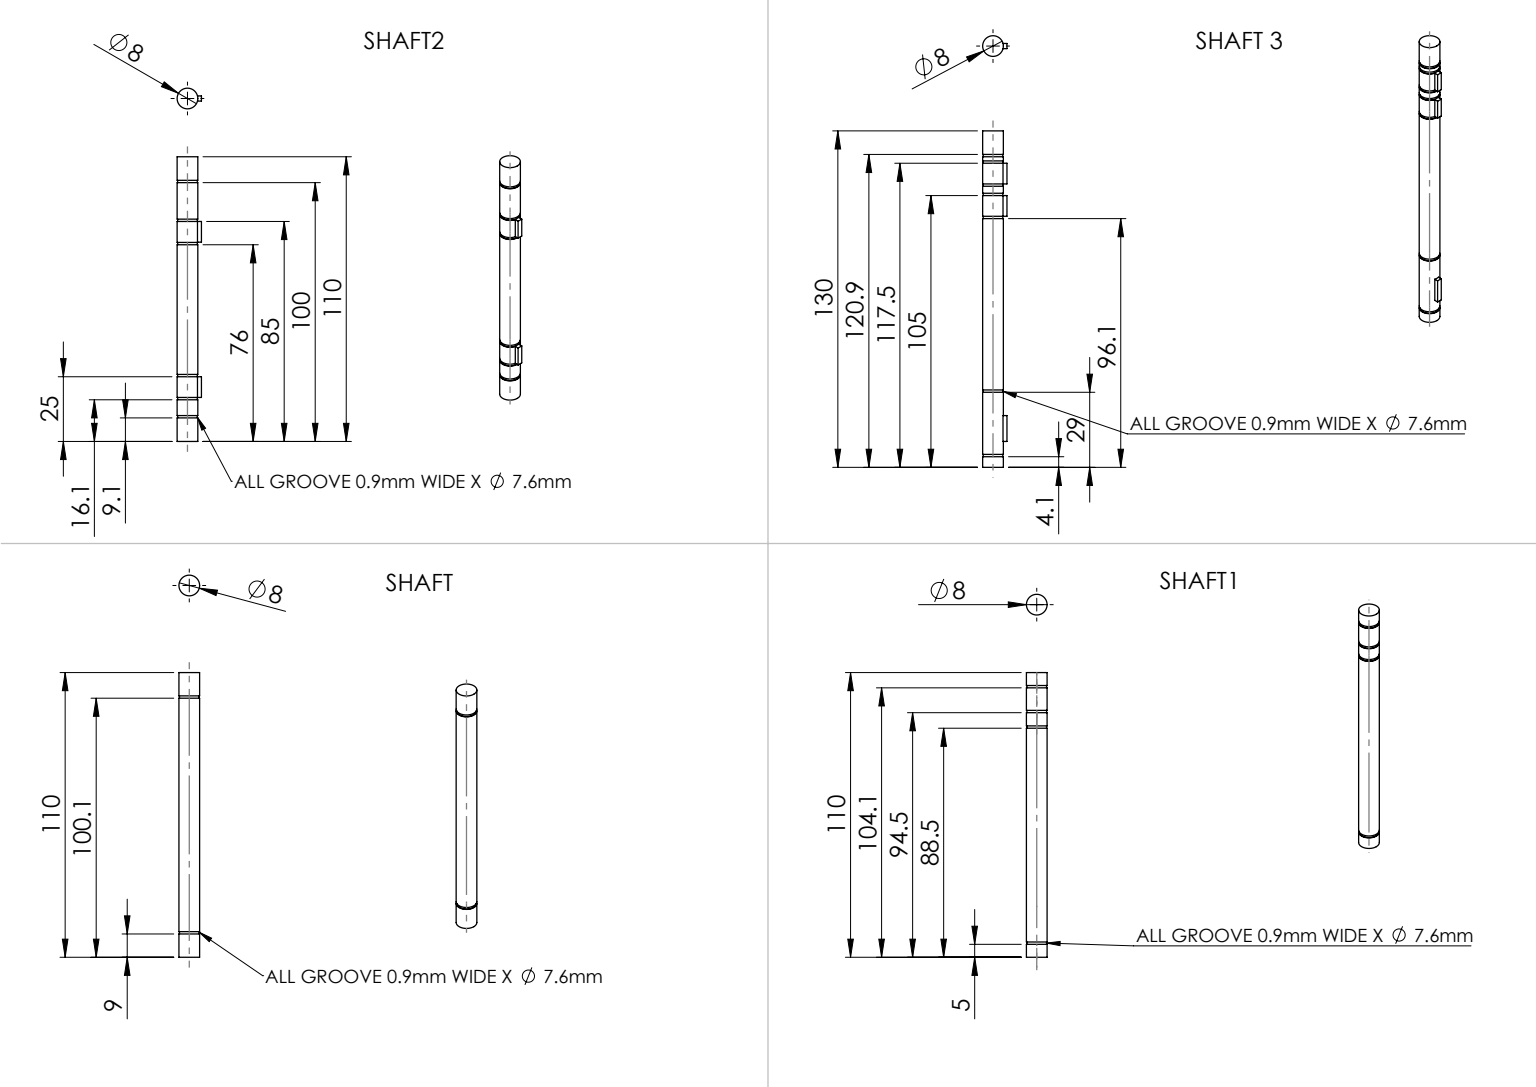
ISO-10303-21;
HEADER;
FILE_DESCRIPTION (('STEP AP214'),
    '1' );
FILE_NAME ('shaft2.step',
    '2026-09-28T15:49:00',
    ( '' ),
    ( '' ),
    'SwSTEP 2.0',
    'SolidWorks 2026',
    '' );
FILE_SCHEMA (( 'AUTOMOTIVE_DESIGN' ));
ENDSEC;

DATA;
#32=ORIENTED_EDGE ( 'NONE', *, *, #23830, .T. ) ;
#40=FACE_OUTER_BOUND ( 'NONE', #7039, .T. ) ;
#47=DIRECTION ( 'NONE',  ( 0.000000000000000000, 0.000000000000000000, -1.000000000000000000 ) ) ;
#82=CARTESIAN_POINT ( 'NONE',  ( -3.799999999999999822, 4.382607293638566128E-16, -21.89999999999999858 ) ) ;
#98=( GEOMETRIC_REPRESENTATION_CONTEXT ( 3 ) GLOBAL_UNCERTAINTY_ASSIGNED_CONTEXT ( ( #24807 ) ) GLOBAL_UNIT_ASSIGNED_CONTEXT ( ( #15841, #16194, #16020 ) ) REPRESENTATION_CONTEXT ( 'NONE', 'WORKASPACE' ) );
#117=DIRECTION ( 'NONE',  ( -1.000000000000000000, 0.000000000000000000, 0.000000000000000000 ) ) ;
#178=CIRCLE ( 'NONE', #22577, 4.000000000000000000 ) ;
#185=VERTEX_POINT ( 'NONE', #4789 ) ;
#210=CARTESIAN_POINT ( 'NONE',  ( 5.400000000000015454, -1.000000000000002220, -22.00000000000000000 ) ) ;
#255=CARTESIAN_POINT ( 'NONE',  ( 0.000000000000000000, -2.710505431213761085E-17, -45.89999999999999858 ) ) ;
#260=ORIENTED_EDGE ( 'NONE', *, *, #3308, .F. ) ;
#266=ORIENTED_EDGE ( 'NONE', *, *, #9713, .F. ) ;
#278=VECTOR ( 'NONE', #10313, 1000.000000000000000 ) ;
#308=ORIENTED_EDGE ( 'NONE', *, *, #26431, .T. ) ;
#342=VERTEX_POINT ( 'NONE', #32678 ) ;
#351=DIRECTION ( 'NONE',  ( -1.000000000000000000, 0.000000000000000000, 0.000000000000000000 ) ) ;
#427=DIRECTION ( 'NONE',  ( 0.000000000000000000, 0.000000000000000000, -1.000000000000000000 ) ) ;
#440=VERTEX_POINT ( 'NONE', #35039 ) ;
#452=ORIENTED_EDGE ( 'NONE', *, *, #14571, .F. ) ;
#462=CARTESIAN_POINT ( 'NONE',  ( 0.000000000000000000, -2.710505431213761085E-17, -21.89999999999999858 ) ) ;
#493=DIRECTION ( 'NONE',  ( 1.000000000000000000, 0.000000000000000000, 0.000000000000000000 ) ) ;
#496=EDGE_CURVE ( 'NONE', #185, #4943, #8530, .T. ) ;
#500=ORIENTED_EDGE ( 'NONE', *, *, #33503, .T. ) ;
#516=FACE_BOUND ( 'NONE', #19608, .T. ) ;
#542=VERTEX_POINT ( 'NONE', #3500 ) ;
#583=DIRECTION ( 'NONE',  ( -1.000000000000000000, 0.000000000000000000, 0.000000000000000000 ) ) ;
#606=CARTESIAN_POINT ( 'NONE',  ( 6.071532165918824830E-15, 1.000000000000000000, 38.00000000000000000 ) ) ;
#619=EDGE_LOOP ( 'NONE', ( #5194, #17904, #27219, #22825 ) ) ;
#628=EDGE_CURVE ( 'NONE', #13726, #1603, #27780, .T. ) ;
#657=EDGE_CURVE ( 'NONE', #5410, #7912, #11948, .T. ) ;
#751=VERTEX_POINT ( 'NONE', #15513 ) ;
#763=DIRECTION ( 'NONE',  ( -0.000000000000000000, 0.000000000000000000, -1.000000000000000000 ) ) ;
#798=DIRECTION ( 'NONE',  ( -1.000000000000000000, 0.000000000000000000, 0.000000000000000000 ) ) ;
#813=PRESENTATION_STYLE_ASSIGNMENT (( #32934 ) ) ;
#825=ORIENTED_EDGE ( 'NONE', *, *, #30231, .F. ) ;
#844=PLANE ( 'NONE',  #8243 ) ;
#853=DIRECTION ( 'NONE',  ( -0.000000000000000000, 0.000000000000000000, -1.000000000000000000 ) ) ;
#880=VECTOR ( 'NONE', #6059, 1000.000000000000000 ) ;
#908=VERTEX_POINT ( 'NONE', #15691 ) ;
#960=LINE ( 'NONE', #1142, #3147 ) ;
#991=CARTESIAN_POINT ( 'NONE',  ( 0.000000000000000000, -2.710505431213761085E-17, 55.00000000000000000 ) ) ;
#1001=VECTOR ( 'NONE', #23243, 1000.000000000000000 ) ;
#1044=ORIENTED_EDGE ( 'NONE', *, *, #17234, .T. ) ;
#1056=CARTESIAN_POINT ( 'NONE',  ( -4.000000000000000000, -2.710505431213761085E-17, -20.99999999999999645 ) ) ;
#1068=ORIENTED_EDGE ( 'NONE', *, *, #2171, .T. ) ;
#1072=ORIENTED_EDGE ( 'NONE', *, *, #10606, .F. ) ;
#1142=CARTESIAN_POINT ( 'NONE',  ( 5.400000000000015454, -1.000000000000002220, 38.00000000000000000 ) ) ;
#1161=ORIENTED_EDGE ( 'NONE', *, *, #13775, .T. ) ;
#1195=ORIENTED_EDGE ( 'NONE', *, *, #24033, .T. ) ;
#1209=DIRECTION ( 'NONE',  ( -1.000000000000000000, 0.000000000000000000, 0.000000000000000000 ) ) ;
#1266=EDGE_LOOP ( 'NONE', ( #9909, #9614 ) ) ;
#1268=CARTESIAN_POINT ( 'NONE',  ( 5.400000000000015454, -1.000000000000002220, 38.00000000000000000 ) ) ;
#1317=VERTEX_POINT ( 'NONE', #31534 ) ;
#1353=UNCERTAINTY_MEASURE_WITH_UNIT (LENGTH_MEASURE( 1.000000000000000082E-05 ), #3538, 'distance_accuracy_value', 'NONE');
#1355=EDGE_LOOP ( 'NONE', ( #23025, #6634 ) ) ;
#1381=ORIENTED_EDGE ( 'NONE', *, *, #35324, .T. ) ;
#1383=CARTESIAN_POINT ( 'NONE',  ( -4.000000000000000000, -2.710505431213761085E-17, -30.00000000000000711 ) ) ;
#1402=DIRECTION ( 'NONE',  ( 0.000000000000000000, 0.000000000000000000, -1.000000000000000000 ) ) ;
#1407=CARTESIAN_POINT ( 'NONE',  ( 0.000000000000000000, -2.710505431213761085E-17, -45.00000000000000000 ) ) ;
#1426=CIRCLE ( 'NONE', #24430, 4.000000000000000000 ) ;
#1443=LINE ( 'NONE', #17456, #9565 ) ;
#1459=AXIS2_PLACEMENT_3D ( 'NONE', #33980, #25881, #34827 ) ;
#1469=ORIENTED_EDGE ( 'NONE', *, *, #628, .F. ) ;
#1480=DIRECTION ( 'NONE',  ( 0.000000000000000000, 0.000000000000000000, -1.000000000000000000 ) ) ;
#1503=FACE_OUTER_BOUND ( 'NONE', #12935, .T. ) ;
#1586=ADVANCED_FACE ( 'NONE', ( #16721, #16553 ), #14543, .T. ) ;
#1589=VECTOR ( 'NONE', #10467, 1000.000000000000000 ) ;
#1590=DIRECTION ( 'NONE',  ( 0.000000000000000000, 0.000000000000000000, 1.000000000000000000 ) ) ;
#1592=LINE ( 'NONE', #20641, #29686 ) ;
#1603=VERTEX_POINT ( 'NONE', #14378 ) ;
#1615=CARTESIAN_POINT ( 'NONE',  ( 0.000000000000000000, -2.710505431213761085E-17, 45.00000000000000000 ) ) ;
#1632=FACE_OUTER_BOUND ( 'NONE', #3397, .T. ) ;
#1636=DIRECTION ( 'NONE',  ( 0.000000000000000000, 0.000000000000000000, -1.000000000000000000 ) ) ;
#1656=VERTEX_POINT ( 'NONE', #24846 ) ;
#1666=AXIS2_PLACEMENT_3D ( 'NONE', #8199, #16112, #18830 ) ;
#1816=CARTESIAN_POINT ( 'NONE',  ( 0.000000000000000000, -2.710505431213761085E-17, 38.90000000000000568 ) ) ;
#1886=AXIS2_PLACEMENT_3D ( 'NONE', #15897, #7452, #7275 ) ;
#1914=DIRECTION ( 'NONE',  ( -0.000000000000000000, 0.000000000000000000, -1.000000000000000000 ) ) ;
#1927=ORIENTED_EDGE ( 'NONE', *, *, #25819, .F. ) ;
#1951=ADVANCED_FACE ( 'NONE', ( #32372, #32541 ), #35096, .F. ) ;
#1972=ORIENTED_EDGE ( 'NONE', *, *, #26406, .F. ) ;
#2019=( NAMED_UNIT ( * ) PLANE_ANGLE_UNIT ( ) SI_UNIT ( $, .RADIAN. ) );
#2103=DIRECTION ( 'NONE',  ( 1.000000000000000000, 0.000000000000000000, 0.000000000000000000 ) ) ;
#2109=DIRECTION ( 'NONE',  ( 1.000000000000000000, 0.000000000000000000, 0.000000000000000000 ) ) ;
#2124=VECTOR ( 'NONE', #11080, 1000.000000000000000 ) ;
#2160=ORIENTED_EDGE ( 'NONE', *, *, #21209, .T. ) ;
#2171=EDGE_CURVE ( 'NONE', #13101, #10171, #22102, .T. ) ;
#2187=CARTESIAN_POINT ( 'NONE',  ( -3.799999999999999822, 4.382607293638566128E-16, 38.00000000000000711 ) ) ;
#2192=DIRECTION ( 'NONE',  ( -1.000000000000000000, 1.110223024625156540E-16, 0.000000000000000000 ) ) ;
#2240=LINE ( 'NONE', #24180, #6682 ) ;
#2272=ORIENTED_EDGE ( 'NONE', *, *, #11488, .F. ) ;
#2281=CARTESIAN_POINT ( 'NONE',  ( 0.000000000000000000, -2.710505431213761085E-17, 45.89999999999999858 ) ) ;
#2288=VERTEX_POINT ( 'NONE', #17558 ) ;
#2313=DIRECTION ( 'NONE',  ( 1.000000000000000000, -1.110223024625156540E-16, 0.000000000000000000 ) ) ;
#2325=CARTESIAN_POINT ( 'NONE',  ( 3.872983346207429900, -1.000000000000003553, -30.00000000000000711 ) ) ;
#2330=VERTEX_POINT ( 'NONE', #28745 ) ;
#2342=EDGE_LOOP ( 'NONE', ( #31787, #21630, #16161, #3142, #11858 ) ) ;
#2389=DIRECTION ( 'NONE',  ( -0.000000000000000000, 0.000000000000000000, -1.000000000000000000 ) ) ;
#2447=EDGE_CURVE ( 'NONE', #26362, #542, #27119, .T. ) ;
#2545=CIRCLE ( 'NONE', #18605, 3.799999999999999822 ) ;
#2556=ORIENTED_EDGE ( 'NONE', *, *, #17988, .F. ) ;
#2559=SHAPE_REPRESENTATION_RELATIONSHIP ( 'NONE' , 'NONE' ,  #5681, #8640 ) ;
#2582=CIRCLE ( 'NONE', #29610, 4.000000000000000000 ) ;
#2638=ORIENTED_EDGE ( 'NONE', *, *, #16294, .T. ) ;
#2640=ORIENTED_EDGE ( 'NONE', *, *, #29026, .T. ) ;
#2644=ORIENTED_EDGE ( 'NONE', *, *, #496, .F. ) ;
#2660=EDGE_CURVE ( 'NONE', #15153, #17557, #13600, .T. ) ;
#2686=CIRCLE ( 'NONE', #22185, 3.799999999999999822 ) ;
#2770=CARTESIAN_POINT ( 'NONE',  ( 0.000000000000000000, -2.710505431213761085E-17, 38.00000000000000711 ) ) ;
#2821=VECTOR ( 'NONE', #6341, 1000.000000000000000 ) ;
#2871=ORIENTED_EDGE ( 'NONE', *, *, #30764, .F. ) ;
#2885=FACE_BOUND ( 'NONE', #33804, .T. ) ;
#2886=DIRECTION ( 'NONE',  ( 0.000000000000000000, 0.000000000000000000, -1.000000000000000000 ) ) ;
#2902=EDGE_LOOP ( 'NONE', ( #9794, #22603, #23283, #8221 ) ) ;
#2907=EDGE_LOOP ( 'NONE', ( #5346, #10050 ) ) ;
#2959=CARTESIAN_POINT ( 'NONE',  ( 3.799999999999999822, 4.382607293638566128E-16, 45.89999999999999858 ) ) ;
#2979=DIRECTION ( 'NONE',  ( 0.000000000000000000, 0.000000000000000000, 1.000000000000000000 ) ) ;
#3015=DIRECTION ( 'NONE',  ( -1.000000000000000000, 1.110223024625156540E-16, 0.000000000000000000 ) ) ;
#3053=ORIENTED_EDGE ( 'NONE', *, *, #8030, .T. ) ;
#3056=DIRECTION ( 'NONE',  ( 0.000000000000000000, 0.000000000000000000, 1.000000000000000000 ) ) ;
#3073=CIRCLE ( 'NONE', #23781, 3.799999999999999822 ) ;
#3142=ORIENTED_EDGE ( 'NONE', *, *, #28661, .T. ) ;
#3147=VECTOR ( 'NONE', #25455, 1000.000000000000000 ) ;
#3151=FACE_OUTER_BOUND ( 'NONE', #30786, .T. ) ;
#3240=ORIENTED_EDGE ( 'NONE', *, *, #31686, .T. ) ;
#3251=ORIENTED_EDGE ( 'NONE', *, *, #9751, .T. ) ;
#3308=EDGE_CURVE ( 'NONE', #13350, #4520, #28897, .T. ) ;
#3310=LINE ( 'NONE', #8861, #35043 ) ;
#3315=CARTESIAN_POINT ( 'NONE',  ( 3.872983346207429900, -1.000000000000003553, 55.00000000000000000 ) ) ;
#3318=CIRCLE ( 'NONE', #23430, 4.000000000000000000 ) ;
#3397=EDGE_LOOP ( 'NONE', ( #19722, #11550, #20094, #1381 ) ) ;
#3437=CARTESIAN_POINT ( 'NONE',  ( 0.000000000000000000, -2.710505431213761085E-17, 55.00000000000000000 ) ) ;
#3452=DIRECTION ( 'NONE',  ( -0.000000000000000000, 0.000000000000000000, -1.000000000000000000 ) ) ;
#3462=VERTEX_POINT ( 'NONE', #30278 ) ;
#3485=ORIENTED_EDGE ( 'NONE', *, *, #23597, .F. ) ;
#3500=CARTESIAN_POINT ( 'NONE',  ( 3.872983346207416133, 1.000000000000001110, -29.99999999999999289 ) ) ;
#3501=ORIENTED_EDGE ( 'NONE', *, *, #30231, .T. ) ;
#3502=CARTESIAN_POINT ( 'NONE',  ( 5.400000000000015454, -1.000000000000002220, 30.00000000000000000 ) ) ;
#3513=EDGE_LOOP ( 'NONE', ( #35507, #10361 ) ) ;
#3529=DIRECTION ( 'NONE',  ( -1.000000000000000000, 0.000000000000000000, 0.000000000000000000 ) ) ;
#3534=DIRECTION ( 'NONE',  ( 0.000000000000000000, 0.000000000000000000, 1.000000000000000000 ) ) ;
#3538=( LENGTH_UNIT ( ) NAMED_UNIT ( * ) SI_UNIT ( .MILLI., .METRE. ) );
#3542=LINE ( 'NONE', #14490, #19352 ) ;
#3566=CARTESIAN_POINT ( 'NONE',  ( 3.799999999999999822, -2.710505431213761085E-17, -30.00000000000000711 ) ) ;
#3582=STYLED_ITEM ( 'NONE', ( #813 ), #22482 ) ;
#3641=DIRECTION ( 'NONE',  ( -0.000000000000000000, 0.000000000000000000, -1.000000000000000000 ) ) ;
#3685=VERTEX_POINT ( 'NONE', #28810 ) ;
#3698=VECTOR ( 'NONE', #15369, 1000.000000000000000 ) ;
#3756=DIRECTION ( 'NONE',  ( 0.000000000000000000, 0.000000000000000000, -1.000000000000000000 ) ) ;
#3779=DIRECTION ( 'NONE',  ( 0.000000000000000000, 0.000000000000000000, -1.000000000000000000 ) ) ;
#3809=ORIENTED_EDGE ( 'NONE', *, *, #6680, .F. ) ;
#3820=VERTEX_POINT ( 'NONE', #18530 ) ;
#3822=LINE ( 'NONE', #31353, #1001 ) ;
#3905=CARTESIAN_POINT ( 'NONE',  ( -3.799999999999999822, 4.382607293638566128E-16, -45.00000000000000000 ) ) ;
#3928=DIRECTION ( 'NONE',  ( -0.000000000000000000, 0.000000000000000000, -1.000000000000000000 ) ) ;
#4014=DIRECTION ( 'NONE',  ( 0.000000000000000000, 0.000000000000000000, -1.000000000000000000 ) ) ;
#4016=DIRECTION ( 'NONE',  ( -1.000000000000000000, 0.000000000000000000, 0.000000000000000000 ) ) ;
#4025=CARTESIAN_POINT ( 'NONE',  ( 0.000000000000000000, -2.710505431213761085E-17, -21.89999999999999858 ) ) ;
#4028=EDGE_CURVE ( 'NONE', #20179, #14725, #27358, .T. ) ;
#4035=EDGE_CURVE ( 'NONE', #31214, #35587, #27806, .T. ) ;
#4078=EDGE_CURVE ( 'NONE', #20179, #3685, #18014, .T. ) ;
#4079=CARTESIAN_POINT ( 'NONE',  ( -3.799999999999999822, 4.382607293638566128E-16, 29.09999999999999787 ) ) ;
#4097=ORIENTED_EDGE ( 'NONE', *, *, #16943, .F. ) ;
#4108=CARTESIAN_POINT ( 'NONE',  ( 0.000000000000000000, -2.710505431213761085E-17, 45.89999999999999858 ) ) ;
#4124=AXIS2_PLACEMENT_3D ( 'NONE', #1615, #29162, #4322 ) ;
#4151=DIRECTION ( 'NONE',  ( 1.000000000000000000, 0.000000000000000000, 0.000000000000000000 ) ) ;
#4182=EDGE_CURVE ( 'NONE', #185, #31659, #32397, .T. ) ;
#4231=VERTEX_POINT ( 'NONE', #27841 ) ;
#4249=CARTESIAN_POINT ( 'NONE',  ( 0.000000000000000000, -2.710505431213761085E-17, 29.09999999999999787 ) ) ;
#4260=CARTESIAN_POINT ( 'NONE',  ( 0.000000000000000000, -2.710505431213761085E-17, 45.89999999999999858 ) ) ;
#4283=EDGE_LOOP ( 'NONE', ( #22004, #17712 ) ) ;
#4322=DIRECTION ( 'NONE',  ( -1.000000000000000000, 0.000000000000000000, 0.000000000000000000 ) ) ;
#4349=FACE_OUTER_BOUND ( 'NONE', #14294, .T. ) ;
#4351=AXIS2_PLACEMENT_3D ( 'NONE', #9477, #20433, #21120 ) ;
#4362=DIRECTION ( 'NONE',  ( -0.000000000000000000, 0.000000000000000000, -1.000000000000000000 ) ) ;
#4406=ORIENTED_EDGE ( 'NONE', *, *, #25529, .F. ) ;
#4408=ADVANCED_FACE ( 'NONE', ( #20596 ), #14482, .T. ) ;
#4411=AXIS2_PLACEMENT_3D ( 'NONE', #1407, #23541, #9853 ) ;
#4418=AXIS2_PLACEMENT_3D ( 'NONE', #18704, #32403, #15636 ) ;
#4426=LINE ( 'NONE', #23492, #3698 ) ;
#4466=ORIENTED_EDGE ( 'NONE', *, *, #8995, .T. ) ;
#4479=CARTESIAN_POINT ( 'NONE',  ( 0.000000000000000000, -2.710505431213761085E-17, 30.00000000000000000 ) ) ;
#4499=ORIENTED_EDGE ( 'NONE', *, *, #12958, .F. ) ;
#4506=EDGE_CURVE ( 'NONE', #26981, #19156, #33949, .T. ) ;
#4507=AXIS2_PLACEMENT_3D ( 'NONE', #25820, #11753, #28152 ) ;
#4508=AXIS2_PLACEMENT_3D ( 'NONE', #30974, #17275, #12610 ) ;
#4520=VERTEX_POINT ( 'NONE', #4079 ) ;
#4553=DIRECTION ( 'NONE',  ( 0.000000000000000000, 0.000000000000000000, -1.000000000000000000 ) ) ;
#4554=DIRECTION ( 'NONE',  ( 1.000000000000000000, 0.000000000000000000, 0.000000000000000000 ) ) ;
#4585=DIRECTION ( 'NONE',  ( -1.000000000000000000, 0.000000000000000000, 0.000000000000000000 ) ) ;
#4628=VERTEX_POINT ( 'NONE', #26379 ) ;
#4635=EDGE_CURVE ( 'NONE', #20295, #16000, #13237, .T. ) ;
#4639=ORIENTED_EDGE ( 'NONE', *, *, #5293, .T. ) ;
#4640=CARTESIAN_POINT ( 'NONE',  ( 5.400000000000015454, -1.000000000000002220, -30.00000000000000000 ) ) ;
#4642=CIRCLE ( 'NONE', #10388, 3.799999999999999822 ) ;
#4659=EDGE_CURVE ( 'NONE', #13726, #9927, #4426, .T. ) ;
#4789=CARTESIAN_POINT ( 'NONE',  ( 3.872983346207429900, -1.000000000000003553, 38.00000000000000711 ) ) ;
#4892=FACE_OUTER_BOUND ( 'NONE', #15777, .T. ) ;
#4906=EDGE_LOOP ( 'NONE', ( #19942, #33349, #3240, #23801 ) ) ;
#4943=VERTEX_POINT ( 'NONE', #1268 ) ;
#4968=CARTESIAN_POINT ( 'NONE',  ( 0.000000000000000000, -2.710505431213761085E-17, 45.00000000000000000 ) ) ;
#4986=CARTESIAN_POINT ( 'NONE',  ( 5.400000000000015454, -1.000000000000002220, -22.00000000000000000 ) ) ;
#5112=DIRECTION ( 'NONE',  ( -1.000000000000000000, 0.000000000000000000, 0.000000000000000000 ) ) ;
#5168=ORIENTED_EDGE ( 'NONE', *, *, #32346, .T. ) ;
#5173=ORIENTED_EDGE ( 'NONE', *, *, #29602, .T. ) ;
#5184=LINE ( 'NONE', #5521, #21124 ) ;
#5190=CYLINDRICAL_SURFACE ( 'NONE', #33155, 4.000000000000000000 ) ;
#5194=ORIENTED_EDGE ( 'NONE', *, *, #657, .F. ) ;
#5219=DIRECTION ( 'NONE',  ( 0.000000000000000000, 0.000000000000000000, 1.000000000000000000 ) ) ;
#5256=FILL_AREA_STYLE_COLOUR ( '', #17344 ) ;
#5274=VECTOR ( 'NONE', #28232, 1000.000000000000000 ) ;
#5284=DIRECTION ( 'NONE',  ( -0.000000000000000000, 0.000000000000000000, -1.000000000000000000 ) ) ;
#5293=EDGE_CURVE ( 'NONE', #6915, #2288, #1426, .T. ) ;
#5315=ORIENTED_EDGE ( 'NONE', *, *, #24033, .F. ) ;
#5323=DIRECTION ( 'NONE',  ( -1.000000000000000000, 1.110223024625156540E-16, 0.000000000000000000 ) ) ;
#5330=ORIENTED_EDGE ( 'NONE', *, *, #496, .T. ) ;
#5346=ORIENTED_EDGE ( 'NONE', *, *, #14740, .F. ) ;
#5410=VERTEX_POINT ( 'NONE', #31478 ) ;
#5413=ORIENTED_EDGE ( 'NONE', *, *, #7663, .F. ) ;
#5450=CYLINDRICAL_SURFACE ( 'NONE', #21036, 3.799999999999999822 ) ;
#5461=ORIENTED_EDGE ( 'NONE', *, *, #28615, .F. ) ;
#5521=CARTESIAN_POINT ( 'NONE',  ( 3.872983346207429900, -1.000000000000003553, 55.00000000000000000 ) ) ;
#5637=VECTOR ( 'NONE', #29723, 1000.000000000000000 ) ;
#5638=CARTESIAN_POINT ( 'NONE',  ( 0.000000000000000000, -2.710505431213761085E-17, -30.00000000000000711 ) ) ;
#5649=ORIENTED_EDGE ( 'NONE', *, *, #25316, .F. ) ;
#5681=SHAPE_REPRESENTATION ( 'shaft2', ( #21307 ), #21360 ) ;
#5696=DIRECTION ( 'NONE',  ( 0.000000000000000000, 0.000000000000000000, 1.000000000000000000 ) ) ;
#5697=DIRECTION ( 'NONE',  ( 0.000000000000000000, 0.000000000000000000, -1.000000000000000000 ) ) ;
#5711=DIRECTION ( 'NONE',  ( -1.000000000000000000, 0.000000000000000000, 0.000000000000000000 ) ) ;
#5713=DIRECTION ( 'NONE',  ( -1.000000000000000000, 0.000000000000000000, 0.000000000000000000 ) ) ;
#5811=ORIENTED_EDGE ( 'NONE', *, *, #17321, .T. ) ;
#5832=CARTESIAN_POINT ( 'NONE',  ( 3.799999999999999822, -2.710505431213761085E-17, 38.00000000000000711 ) ) ;
#5840=DIRECTION ( 'NONE',  ( 0.000000000000000000, 0.000000000000000000, -1.000000000000000000 ) ) ;
#5841=DIRECTION ( 'NONE',  ( 0.000000000000000000, 0.000000000000000000, 1.000000000000000000 ) ) ;
#5854=VERTEX_POINT ( 'NONE', #17912 ) ;
#5871=AXIS2_PLACEMENT_3D ( 'NONE', #19524, #27302, #22064 ) ;
#5899=EDGE_LOOP ( 'NONE', ( #19959, #4466, #24029, #2272 ) ) ;
#5920=ORIENTED_EDGE ( 'NONE', *, *, #30074, .T. ) ;
#5943=DIRECTION ( 'NONE',  ( -0.000000000000000000, 0.000000000000000000, -1.000000000000000000 ) ) ;
#6002=ADVANCED_FACE ( 'NONE', ( #6231, #22779 ), #7114, .T. ) ;
#6012=CARTESIAN_POINT ( 'NONE',  ( 0.000000000000000000, -1.000000000000001554, 38.00000000000000000 ) ) ;
#6014=DIRECTION ( 'NONE',  ( 0.000000000000000000, 0.000000000000000000, 1.000000000000000000 ) ) ;
#6016=DIRECTION ( 'NONE',  ( -1.000000000000000000, 0.000000000000000000, 0.000000000000000000 ) ) ;
#6059=DIRECTION ( 'NONE',  ( -0.000000000000000000, 0.000000000000000000, -1.000000000000000000 ) ) ;
#6078=ADVANCED_FACE ( 'NONE', ( #10181 ), #15555, .T. ) ;
#6094=DIRECTION ( 'NONE',  ( -1.000000000000000000, 0.000000000000000000, 0.000000000000000000 ) ) ;
#6190=DIRECTION ( 'NONE',  ( -1.000000000000000000, 0.000000000000000000, 0.000000000000000000 ) ) ;
#6214=EDGE_CURVE ( 'NONE', #6339, #17196, #14686, .T. ) ;
#6231=FACE_BOUND ( 'NONE', #11676, .T. ) ;
#6265=CARTESIAN_POINT ( 'NONE',  ( -4.000000000000000000, -2.710505431213761085E-17, 55.00000000000000000 ) ) ;
#6270=CARTESIAN_POINT ( 'NONE',  ( 4.000000000000000000, 4.627536653468036720E-16, 38.90000000000000568 ) ) ;
#6334=EDGE_CURVE ( 'NONE', #26981, #19072, #16411, .T. ) ;
#6339=VERTEX_POINT ( 'NONE', #11419 ) ;
#6341=DIRECTION ( 'NONE',  ( 0.000000000000000000, 0.000000000000000000, -1.000000000000000000 ) ) ;
#6359=CARTESIAN_POINT ( 'NONE',  ( 0.000000000000000000, -2.710505431213761085E-17, -21.89999999999999858 ) ) ;
#6361=CARTESIAN_POINT ( 'NONE',  ( 5.400000000000015454, -1.000000000000002220, -22.00000000000000000 ) ) ;
#6363=ADVANCED_FACE ( 'NONE', ( #22383 ), #25281, .T. ) ;
#6402=DIRECTION ( 'NONE',  ( 1.000000000000000000, -1.110223024625156540E-16, 0.000000000000000000 ) ) ;
#6480=DIRECTION ( 'NONE',  ( -1.000000000000000000, 0.000000000000000000, 0.000000000000000000 ) ) ;
#6536=DIRECTION ( 'NONE',  ( 0.000000000000000000, 0.000000000000000000, -1.000000000000000000 ) ) ;
#6593=SHAPE_DEFINITION_REPRESENTATION ( #20122, #5681 ) ;
#6613=DIRECTION ( 'NONE',  ( -1.000000000000000000, 0.000000000000000000, 0.000000000000000000 ) ) ;
#6634=ORIENTED_EDGE ( 'NONE', *, *, #9173, .T. ) ;
#6680=EDGE_CURVE ( 'NONE', #16000, #2330, #2240, .T. ) ;
#6682=VECTOR ( 'NONE', #35175, 1000.000000000000000 ) ;
#6698=ORIENTED_EDGE ( 'NONE', *, *, #24435, .T. ) ;
#6724=AXIS2_PLACEMENT_3D ( 'NONE', #30154, #27468, #7640 ) ;
#6726=ADVANCED_FACE ( 'NONE', ( #40 ), #5450, .T. ) ;
#6762=ORIENTED_EDGE ( 'NONE', *, *, #3308, .T. ) ;
#6764=AXIS2_PLACEMENT_3D ( 'NONE', #15950, #13279, #21519 ) ;
#6791=CARTESIAN_POINT ( 'NONE',  ( -3.799999999999999822, 4.382607293638566128E-16, -30.00000000000000711 ) ) ;
#6811=EDGE_CURVE ( 'NONE', #4231, #34564, #23945, .T. ) ;
#6823=EDGE_CURVE ( 'NONE', #31834, #19156, #19284, .T. ) ;
#6833=LINE ( 'NONE', #26469, #12038 ) ;
#6846=ORIENTED_EDGE ( 'NONE', *, *, #33935, .F. ) ;
#6866=EDGE_LOOP ( 'NONE', ( #3485, #23747, #12315, #18680 ) ) ;
#6872=ORIENTED_EDGE ( 'NONE', *, *, #10606, .T. ) ;
#6901=EDGE_LOOP ( 'NONE', ( #17611, #4639, #24134, #32203 ) ) ;
#6915=VERTEX_POINT ( 'NONE', #28294 ) ;
#6939=DIRECTION ( 'NONE',  ( -1.000000000000000000, 0.000000000000000000, 0.000000000000000000 ) ) ;
#6940=DIRECTION ( 'NONE',  ( -1.000000000000000000, 0.000000000000000000, 0.000000000000000000 ) ) ;
#6982=ADVANCED_FACE ( 'NONE', ( #14585 ), #28654, .T. ) ;
#7039=EDGE_LOOP ( 'NONE', ( #1927, #21556, #20255, #30611 ) ) ;
#7061=VECTOR ( 'NONE', #35344, 1000.000000000000000 ) ;
#7114=PLANE ( 'NONE',  #33118 ) ;
#7169=EDGE_LOOP ( 'NONE', ( #12979, #6872 ) ) ;
#7219=CARTESIAN_POINT ( 'NONE',  ( 3.872983346207416133, 1.000000000000001110, 30.00000000000000000 ) ) ;
#7231=CARTESIAN_POINT ( 'NONE',  ( 0.000000000000000000, -2.710505431213761085E-17, 38.00000000000000711 ) ) ;
#7238=CIRCLE ( 'NONE', #23326, 4.000000000000000000 ) ;
#7258=ADVANCED_FACE ( 'NONE', ( #4349 ), #15297, .T. ) ;
#7275=DIRECTION ( 'NONE',  ( -1.000000000000000000, 0.000000000000000000, 0.000000000000000000 ) ) ;
#7360=EDGE_CURVE ( 'NONE', #8438, #10152, #12475, .T. ) ;
#7452=DIRECTION ( 'NONE',  ( 0.000000000000000000, 0.000000000000000000, -1.000000000000000000 ) ) ;
#7472=DIRECTION ( 'NONE',  ( 1.000000000000000000, 0.000000000000000000, 0.000000000000000000 ) ) ;
#7482=FACE_BOUND ( 'NONE', #19426, .T. ) ;
#7483=CARTESIAN_POINT ( 'NONE',  ( 3.872983346207416133, 1.000000000000001110, 55.00000000000000000 ) ) ;
#7557=CARTESIAN_POINT ( 'NONE',  ( 6.071532165918824830E-15, 1.000000000000000000, -22.00000000000000000 ) ) ;
#7579=ORIENTED_EDGE ( 'NONE', *, *, #26743, .T. ) ;
#7630=AXIS2_PLACEMENT_3D ( 'NONE', #6359, #427, #6190 ) ;
#7638=LINE ( 'NONE', #16260, #15909 ) ;
#7640=DIRECTION ( 'NONE',  ( -1.000000000000000000, 0.000000000000000000, 0.000000000000000000 ) ) ;
#7641=DIRECTION ( 'NONE',  ( 0.000000000000000000, 0.000000000000000000, -1.000000000000000000 ) ) ;
#7663=EDGE_CURVE ( 'NONE', #185, #20179, #19829, .T. ) ;
#7705=ORIENTED_EDGE ( 'NONE', *, *, #18288, .F. ) ;
#7712=ORIENTED_EDGE ( 'NONE', *, *, #4182, .F. ) ;
#7775=AXIS2_PLACEMENT_3D ( 'NONE', #7557, #15815, #2192 ) ;
#7871=ORIENTED_EDGE ( 'NONE', *, *, #22097, .F. ) ;
#7875=DIRECTION ( 'NONE',  ( -0.000000000000000000, 0.000000000000000000, -1.000000000000000000 ) ) ;
#7890=PLANE ( 'NONE',  #19164 ) ;
#7912=VERTEX_POINT ( 'NONE', #6791 ) ;
#7934=DIRECTION ( 'NONE',  ( -1.000000000000000000, 0.000000000000000000, 0.000000000000000000 ) ) ;
#7943=ADVANCED_FACE ( 'NONE', ( #16296 ), #19019, .T. ) ;
#7947=DIRECTION ( 'NONE',  ( -1.000000000000000000, 0.000000000000000000, 0.000000000000000000 ) ) ;
#7957=CARTESIAN_POINT ( 'NONE',  ( 3.799999999999999822, -2.710505431213761085E-17, -30.90000000000000568 ) ) ;
#7976=AXIS2_PLACEMENT_3D ( 'NONE', #13009, #25667, #9442 ) ;
#8030=EDGE_CURVE ( 'NONE', #13101, #26981, #5184, .T. ) ;
#8047=EDGE_CURVE ( 'NONE', #11561, #19855, #21893, .T. ) ;
#8062=PRODUCT_CONTEXT ( 'NONE', #12385, 'mechanical' ) ;
#8144=EDGE_LOOP ( 'NONE', ( #30816, #21870, #34875, #29555 ) ) ;
#8165=DIRECTION ( 'NONE',  ( 0.000000000000000000, 0.000000000000000000, -1.000000000000000000 ) ) ;
#8182=FACE_OUTER_BOUND ( 'NONE', #12820, .T. ) ;
#8194=EDGE_CURVE ( 'NONE', #32016, #14718, #1443, .T. ) ;
#8199=CARTESIAN_POINT ( 'NONE',  ( 0.000000000000000000, -2.710505431213761085E-17, 55.00000000000000000 ) ) ;
#8202=CYLINDRICAL_SURFACE ( 'NONE', #5871, 3.799999999999999822 ) ;
#8221=ORIENTED_EDGE ( 'NONE', *, *, #8194, .F. ) ;
#8228=ORIENTED_EDGE ( 'NONE', *, *, #29602, .F. ) ;
#8243=AXIS2_PLACEMENT_3D ( 'NONE', #28057, #22448, #11479 ) ;
#8263=ORIENTED_EDGE ( 'NONE', *, *, #31691, .T. ) ;
#8278=VERTEX_POINT ( 'NONE', #12423 ) ;
#8309=DIRECTION ( 'NONE',  ( -1.000000000000000000, 0.000000000000000000, 0.000000000000000000 ) ) ;
#8314=EDGE_LOOP ( 'NONE', ( #5168, #3251 ) ) ;
#8347=CARTESIAN_POINT ( 'NONE',  ( 0.000000000000000000, -2.710505431213761085E-17, -55.00000000000000000 ) ) ;
#8352=EDGE_CURVE ( 'NONE', #8849, #29301, #22787, .T. ) ;
#8360=EDGE_LOOP ( 'NONE', ( #16899, #29006, #18947, #21415 ) ) ;
#8366=CIRCLE ( 'NONE', #29644, 3.799999999999999822 ) ;
#8413=DIRECTION ( 'NONE',  ( 0.000000000000000000, 0.000000000000000000, 1.000000000000000000 ) ) ;
#8438=VERTEX_POINT ( 'NONE', #2187 ) ;
#8464=AXIS2_PLACEMENT_3D ( 'NONE', #21684, #24760, #19159 ) ;
#8477=ADVANCED_FACE ( 'NONE', ( #1632 ), #29360, .T. ) ;
#8507=VERTEX_POINT ( 'NONE', #23586 ) ;
#8519=CARTESIAN_POINT ( 'NONE',  ( 3.872983346207416133, 1.000000000000001110, 38.00000000000000000 ) ) ;
#8530=LINE ( 'NONE', #6012, #30066 ) ;
#8542=CARTESIAN_POINT ( 'NONE',  ( 3.799999999999999822, -2.710505431213761085E-17, 30.00000000000000000 ) ) ;
#8565=CARTESIAN_POINT ( 'NONE',  ( 0.000000000000000000, -1.000000000000001554, 38.00000000000000000 ) ) ;
#8640=ADVANCED_BREP_SHAPE_REPRESENTATION ( '', ( #22482, #21307 ), #21360 ) ;
#8703=CARTESIAN_POINT ( 'NONE',  ( 0.000000000000000000, -2.710505431213761085E-17, -30.00000000000000711 ) ) ;
#8723=CARTESIAN_POINT ( 'NONE',  ( 3.799999999999999822, -2.710505431213761085E-17, -45.89999999999999858 ) ) ;
#8773=AXIS2_PLACEMENT_3D ( 'NONE', #25824, #5840, #14279 ) ;
#8793=FACE_OUTER_BOUND ( 'NONE', #14540, .T. ) ;
#8797=VERTEX_POINT ( 'NONE', #1056 ) ;
#8814=ORIENTED_EDGE ( 'NONE', *, *, #21209, .F. ) ;
#8823=CARTESIAN_POINT ( 'NONE',  ( -4.000000000000000000, -2.710505431213761085E-17, 55.00000000000000000 ) ) ;
#8849=VERTEX_POINT ( 'NONE', #17769 ) ;
#8861=CARTESIAN_POINT ( 'NONE',  ( 3.872983346207416133, 1.000000000000001110, 55.00000000000000000 ) ) ;
#8874=DIRECTION ( 'NONE',  ( 0.000000000000000000, 0.000000000000000000, -1.000000000000000000 ) ) ;
#8878=CARTESIAN_POINT ( 'NONE',  ( -4.000000000000000000, -2.710505431213761085E-17, 55.00000000000000000 ) ) ;
#8920=CIRCLE ( 'NONE', #35395, 4.000000000000000000 ) ;
#8945=ORIENTED_EDGE ( 'NONE', *, *, #6811, .F. ) ;
#8975=DIRECTION ( 'NONE',  ( -1.000000000000000000, 0.000000000000000000, 0.000000000000000000 ) ) ;
#8995=EDGE_CURVE ( 'NONE', #6915, #6339, #23539, .T. ) ;
#9029=AXIS2_PLACEMENT_3D ( 'NONE', #5638, #47, #8309 ) ;
#9047=AXIS2_PLACEMENT_3D ( 'NONE', #8565, #35250, #3015 ) ;
#9056=AXIS2_PLACEMENT_3D ( 'NONE', #9069, #6536, #6016 ) ;
#9061=FACE_OUTER_BOUND ( 'NONE', #11005, .T. ) ;
#9067=CARTESIAN_POINT ( 'NONE',  ( 0.000000000000000000, -2.710505431213761085E-17, 45.00000000000000000 ) ) ;
#9069=CARTESIAN_POINT ( 'NONE',  ( 0.000000000000000000, -2.710505431213761085E-17, -20.99999999999999645 ) ) ;
#9072=CARTESIAN_POINT ( 'NONE',  ( 5.400000000000015454, -1.000000000000002220, 30.00000000000000000 ) ) ;
#9096=ADVANCED_FACE ( 'NONE', ( #30541 ), #13454, .F. ) ;
#9104=( NAMED_UNIT ( * ) SI_UNIT ( $, .STERADIAN. ) SOLID_ANGLE_UNIT ( ) );
#9125=FACE_BOUND ( 'NONE', #28178, .T. ) ;
#9128=DIRECTION ( 'NONE',  ( 0.000000000000000000, 0.000000000000000000, -1.000000000000000000 ) ) ;
#9138=CARTESIAN_POINT ( 'NONE',  ( 6.071532165918824830E-15, 1.000000000000000000, -30.00000000000000000 ) ) ;
#9141=LINE ( 'NONE', #6265, #24937 ) ;
#9173=EDGE_CURVE ( 'NONE', #12368, #32016, #21689, .T. ) ;
#9245=PLANE ( 'NONE',  #11658 ) ;
#9276=CARTESIAN_POINT ( 'NONE',  ( 0.000000000000000000, -1.000000000000001554, -30.00000000000000000 ) ) ;
#9293=VECTOR ( 'NONE', #9128, 1000.000000000000000 ) ;
#9374=ORIENTED_EDGE ( 'NONE', *, *, #4078, .F. ) ;
#9412=DIRECTION ( 'NONE',  ( 1.000000000000000000, 0.000000000000000000, 0.000000000000000000 ) ) ;
#9427=EDGE_LOOP ( 'NONE', ( #12031, #25587, #5461, #7871 ) ) ;
#9442=DIRECTION ( 'NONE',  ( -1.000000000000000000, 0.000000000000000000, 0.000000000000000000 ) ) ;
#9477=CARTESIAN_POINT ( 'NONE',  ( 0.000000000000000000, -2.710505431213761085E-17, 38.00000000000000711 ) ) ;
#9497=ADVANCED_FACE ( 'NONE', ( #9061 ), #20019, .T. ) ;
#9565=VECTOR ( 'NONE', #28280, 1000.000000000000000 ) ;
#9574=ADVANCED_FACE ( 'NONE', ( #17147 ), #22552, .T. ) ;
#9614=ORIENTED_EDGE ( 'NONE', *, *, #29338, .T. ) ;
#9631=DIRECTION ( 'NONE',  ( 0.000000000000000000, 0.000000000000000000, -1.000000000000000000 ) ) ;
#9661=AXIS2_PLACEMENT_3D ( 'NONE', #28427, #14026, #14542 ) ;
#9683=CARTESIAN_POINT ( 'NONE',  ( 4.000000000000000000, 4.627536653468036720E-16, 55.00000000000000000 ) ) ;
#9713=EDGE_CURVE ( 'NONE', #15438, #342, #25987, .T. ) ;
#9751=EDGE_CURVE ( 'NONE', #25349, #26576, #25175, .T. ) ;
#9772=DIRECTION ( 'NONE',  ( -0.000000000000000000, 0.000000000000000000, -1.000000000000000000 ) ) ;
#9773=CARTESIAN_POINT ( 'NONE',  ( 0.000000000000000000, -2.710505431213761085E-17, 29.09999999999999787 ) ) ;
#9794=ORIENTED_EDGE ( 'NONE', *, *, #9173, .F. ) ;
#9806=PRODUCT ( 'shaft2', 'shaft2', '', ( #8062 ) ) ;
#9852=CARTESIAN_POINT ( 'NONE',  ( 0.000000000000000000, -2.710505431213761085E-17, -45.89999999999999858 ) ) ;
#9853=DIRECTION ( 'NONE',  ( -1.000000000000000000, 0.000000000000000000, 0.000000000000000000 ) ) ;
#9877=CARTESIAN_POINT ( 'NONE',  ( 3.799999999999999822, -2.710505431213761085E-17, 38.90000000000000568 ) ) ;
#9908=CARTESIAN_POINT ( 'NONE',  ( -4.000000000000000000, -2.710505431213761085E-17, 38.90000000000000568 ) ) ;
#9909=ORIENTED_EDGE ( 'NONE', *, *, #25316, .T. ) ;
#9927=VERTEX_POINT ( 'NONE', #24353 ) ;
#9934=CARTESIAN_POINT ( 'NONE',  ( 0.000000000000000000, 0.000000000000000000, -22.00000000000000000 ) ) ;
#10050=ORIENTED_EDGE ( 'NONE', *, *, #6214, .F. ) ;
#10080=PLANE ( 'NONE',  #29070 ) ;
#10136=DIRECTION ( 'NONE',  ( -0.000000000000000000, 0.000000000000000000, -1.000000000000000000 ) ) ;
#10152=VERTEX_POINT ( 'NONE', #11546 ) ;
#10171=VERTEX_POINT ( 'NONE', #15246 ) ;
#10181=FACE_OUTER_BOUND ( 'NONE', #1266, .T. ) ;
#10183=DIRECTION ( 'NONE',  ( -1.000000000000000000, 0.000000000000000000, 0.000000000000000000 ) ) ;
#10232=EDGE_LOOP ( 'NONE', ( #266, #5649, #2640, #1072 ) ) ;
#10254=VERTEX_POINT ( 'NONE', #15776 ) ;
#10273=FACE_OUTER_BOUND ( 'NONE', #4906, .T. ) ;
#10280=AXIS2_PLACEMENT_3D ( 'NONE', #17181, #9631, #3529 ) ;
#10290=DIRECTION ( 'NONE',  ( -1.000000000000000000, 0.000000000000000000, 0.000000000000000000 ) ) ;
#10313=DIRECTION ( 'NONE',  ( -0.000000000000000000, 0.000000000000000000, -1.000000000000000000 ) ) ;
#10314=ORIENTED_EDGE ( 'NONE', *, *, #24298, .F. ) ;
#10355=PRODUCT_DEFINITION_FORMATION_WITH_SPECIFIED_SOURCE ( 'ANY', '', #9806, .NOT_KNOWN. ) ;
#10361=ORIENTED_EDGE ( 'NONE', *, *, #25562, .F. ) ;
#10388=AXIS2_PLACEMENT_3D ( 'NONE', #15836, #29730, #26855 ) ;
#10467=DIRECTION ( 'NONE',  ( -0.000000000000000000, 0.000000000000000000, -1.000000000000000000 ) ) ;
#10534=CARTESIAN_POINT ( 'NONE',  ( 0.000000000000000000, -2.710505431213761085E-17, 55.00000000000000000 ) ) ;
#10567=DIRECTION ( 'NONE',  ( -0.000000000000000000, 0.000000000000000000, -1.000000000000000000 ) ) ;
#10573=EDGE_CURVE ( 'NONE', #21964, #19855, #23006, .T. ) ;
#10606=EDGE_CURVE ( 'NONE', #342, #8507, #11528, .T. ) ;
#10723=DIRECTION ( 'NONE',  ( 1.000000000000000000, 0.000000000000000000, 0.000000000000000000 ) ) ;
#10747=CARTESIAN_POINT ( 'NONE',  ( -3.799999999999999822, -2.710505431213761085E-17, 45.89999999999999858 ) ) ;
#10767=UNCERTAINTY_MEASURE_WITH_UNIT (LENGTH_MEASURE( 1.000000000000000082E-05 ), #34242, 'distance_accuracy_value', 'NONE');
#10786=FACE_BOUND ( 'NONE', #25248, .T. ) ;
#10820=EDGE_CURVE ( 'NONE', #2288, #6915, #19009, .T. ) ;
#11005=EDGE_LOOP ( 'NONE', ( #17824, #22868, #33564, #20176 ) ) ;
#11040=EDGE_LOOP ( 'NONE', ( #2644, #31547, #19899, #10314 ) ) ;
#11080=DIRECTION ( 'NONE',  ( 0.000000000000000000, 0.000000000000000000, 1.000000000000000000 ) ) ;
#11082=CARTESIAN_POINT ( 'NONE',  ( 0.000000000000000000, -2.710505431213761085E-17, 38.00000000000000711 ) ) ;
#11145=DIRECTION ( 'NONE',  ( 1.000000000000000000, -1.110223024625156540E-16, 0.000000000000000000 ) ) ;
#11219=EDGE_CURVE ( 'NONE', #5854, #908, #17267, .T. ) ;
#11242=DIRECTION ( 'NONE',  ( 0.000000000000000000, 0.000000000000000000, -1.000000000000000000 ) ) ;
#11277=CARTESIAN_POINT ( 'NONE',  ( 0.000000000000000000, -2.710505431213761085E-17, 29.09999999999999787 ) ) ;
#11328=DIRECTION ( 'NONE',  ( 1.000000000000000000, 0.000000000000000000, 0.000000000000000000 ) ) ;
#11354=ORIENTED_EDGE ( 'NONE', *, *, #28766, .F. ) ;
#11419=CARTESIAN_POINT ( 'NONE',  ( 4.000000000000000000, 4.627536653468036720E-16, -55.00000000000000000 ) ) ;
#11479=DIRECTION ( 'NONE',  ( 1.000000000000000000, 0.000000000000000000, 0.000000000000000000 ) ) ;
#11488=EDGE_CURVE ( 'NONE', #2288, #17196, #31169, .T. ) ;
#11495=PLANE ( 'NONE',  #14361 ) ;
#11528=CIRCLE ( 'NONE', #32225, 4.000000000000000000 ) ;
#11546=CARTESIAN_POINT ( 'NONE',  ( 3.799999999999999822, -2.710505431213761085E-17, 38.00000000000000711 ) ) ;
#11550=ORIENTED_EDGE ( 'NONE', *, *, #17150, .F. ) ;
#11555=AXIS2_PLACEMENT_3D ( 'NONE', #3437, #5943, #14385 ) ;
#11561=VERTEX_POINT ( 'NONE', #25954 ) ;
#11619=CARTESIAN_POINT ( 'NONE',  ( 0.000000000000000000, -2.710505431213761085E-17, -30.90000000000000568 ) ) ;
#11621=LINE ( 'NONE', #33588, #28007 ) ;
#11626=DIRECTION ( 'NONE',  ( 0.000000000000000000, 0.000000000000000000, -1.000000000000000000 ) ) ;
#11658=AXIS2_PLACEMENT_3D ( 'NONE', #6361, #33210, #6014 ) ;
#11660=CARTESIAN_POINT ( 'NONE',  ( 0.000000000000000000, -2.710505431213761085E-17, 38.90000000000000568 ) ) ;
#11674=EDGE_CURVE ( 'NONE', #542, #3462, #17402, .T. ) ;
#11676=EDGE_LOOP ( 'NONE', ( #6846, #31793 ) ) ;
#11753=DIRECTION ( 'NONE',  ( -0.000000000000000000, 0.000000000000000000, -1.000000000000000000 ) ) ;
#11829=AXIS2_PLACEMENT_3D ( 'NONE', #27477, #27291, #10723 ) ;
#11840=CARTESIAN_POINT ( 'NONE',  ( 0.000000000000000000, -2.710505431213761085E-17, 55.00000000000000000 ) ) ;
#11858=ORIENTED_EDGE ( 'NONE', *, *, #26431, .F. ) ;
#11898=VECTOR ( 'NONE', #29313, 1000.000000000000000 ) ;
#11926=PRODUCT_DEFINITION_CONTEXT ( 'detailed design', #17894, 'design' ) ;
#11948=LINE ( 'NONE', #17506, #31206 ) ;
#11978=CARTESIAN_POINT ( 'NONE',  ( -3.799999999999999822, -2.710505431213761085E-17, 45.00000000000000000 ) ) ;
#12017=DIRECTION ( 'NONE',  ( -1.000000000000000000, 0.000000000000000000, 0.000000000000000000 ) ) ;
#12031=ORIENTED_EDGE ( 'NONE', *, *, #18572, .T. ) ;
#12038=VECTOR ( 'NONE', #12057, 1000.000000000000000 ) ;
#12057=DIRECTION ( 'NONE',  ( 0.000000000000000000, 0.000000000000000000, 1.000000000000000000 ) ) ;
#12069=EDGE_LOOP ( 'NONE', ( #29502, #26685, #15598, #20219, #14461, #1068 ) ) ;
#12085=EDGE_CURVE ( 'NONE', #19855, #21964, #23081, .T. ) ;
#12146=VECTOR ( 'NONE', #3641, 1000.000000000000000 ) ;
#12228=EDGE_LOOP ( 'NONE', ( #35230, #260, #21912, #1195 ) ) ;
#12272=AXIS2_PLACEMENT_3D ( 'NONE', #12378, #1402, #6613 ) ;
#12305=CARTESIAN_POINT ( 'NONE',  ( 0.000000000000000000, -2.710505431213761085E-17, -55.00000000000000000 ) ) ;
#12315=ORIENTED_EDGE ( 'NONE', *, *, #15009, .T. ) ;
#12341=DIRECTION ( 'NONE',  ( 0.000000000000000000, 0.000000000000000000, -1.000000000000000000 ) ) ;
#12368=VERTEX_POINT ( 'NONE', #16291 ) ;
#12378=CARTESIAN_POINT ( 'NONE',  ( 0.000000000000000000, -2.710505431213761085E-17, 30.00000000000000000 ) ) ;
#12385=APPLICATION_CONTEXT ( 'automotive_design' ) ;
#12411=FACE_OUTER_BOUND ( 'NONE', #6866, .T. ) ;
#12423=CARTESIAN_POINT ( 'NONE',  ( -4.000000000000000000, -2.710505431213761085E-17, -45.00000000000000000 ) ) ;
#12475=CIRCLE ( 'NONE', #28591, 3.799999999999999822 ) ;
#12549=CARTESIAN_POINT ( 'NONE',  ( 5.400000000000003020, 1.000000000000000888, -22.00000000000000000 ) ) ;
#12610=DIRECTION ( 'NONE',  ( -1.000000000000000000, 0.000000000000000000, 0.000000000000000000 ) ) ;
#12707=DIRECTION ( 'NONE',  ( -1.000000000000000000, 0.000000000000000000, 0.000000000000000000 ) ) ;
#12725=DIRECTION ( 'NONE',  ( 0.000000000000000000, 0.000000000000000000, 1.000000000000000000 ) ) ;
#12820=EDGE_LOOP ( 'NONE', ( #25504, #22788, #31334, #14223 ) ) ;
#12826=DIRECTION ( 'NONE',  ( -1.000000000000000000, 0.000000000000000000, 0.000000000000000000 ) ) ;
#12836=ADVANCED_FACE ( 'NONE', ( #25195, #516 ), #11495, .F. ) ;
#12849=VECTOR ( 'NONE', #30351, 1000.000000000000000 ) ;
#12861=FACE_OUTER_BOUND ( 'NONE', #29147, .T. ) ;
#12866=AXIS2_PLACEMENT_3D ( 'NONE', #21850, #8165, #19145 ) ;
#12924=CARTESIAN_POINT ( 'NONE',  ( 3.872983346207429900, -1.000000000000003553, -22.00000000000000000 ) ) ;
#12935=EDGE_LOOP ( 'NONE', ( #8814, #3053, #16993, #16322 ) ) ;
#12958=EDGE_CURVE ( 'NONE', #440, #1656, #14388, .T. ) ;
#12979=ORIENTED_EDGE ( 'NONE', *, *, #20850, .T. ) ;
#12992=PRESENTATION_STYLE_ASSIGNMENT (( #32781 ) ) ;
#13002=VECTOR ( 'NONE', #14620, 1000.000000000000000 ) ;
#13009=CARTESIAN_POINT ( 'NONE',  ( 0.000000000000000000, -2.710505431213761085E-17, 55.00000000000000000 ) ) ;
#13046=ADVANCED_FACE ( 'NONE', ( #15239 ), #26976, .T. ) ;
#13064=DIRECTION ( 'NONE',  ( 1.000000000000000000, -1.110223024625156540E-16, 0.000000000000000000 ) ) ;
#13101=VERTEX_POINT ( 'NONE', #12924 ) ;
#13165=CIRCLE ( 'NONE', #26365, 4.000000000000000000 ) ;
#13237=LINE ( 'NONE', #18259, #16874 ) ;
#13273=ADVANCED_FACE ( 'NONE', ( #35604, #16128 ), #22076, .F. ) ;
#13279=DIRECTION ( 'NONE',  ( 0.000000000000000000, 0.000000000000000000, -1.000000000000000000 ) ) ;
#13288=CARTESIAN_POINT ( 'NONE',  ( 0.000000000000000000, -2.710505431213761085E-17, 55.00000000000000000 ) ) ;
#13350=VERTEX_POINT ( 'NONE', #22591 ) ;
#13351=CARTESIAN_POINT ( 'NONE',  ( 0.000000000000000000, -2.710505431213761085E-17, 55.00000000000000000 ) ) ;
#13376=DIRECTION ( 'NONE',  ( 1.000000000000000000, 0.000000000000000000, 0.000000000000000000 ) ) ;
#13399=VECTOR ( 'NONE', #33911, 1000.000000000000000 ) ;
#13438=AXIS2_PLACEMENT_3D ( 'NONE', #11660, #30414, #25190 ) ;
#13447=DIRECTION ( 'NONE',  ( -1.000000000000000000, 0.000000000000000000, 0.000000000000000000 ) ) ;
#13454=PLANE ( 'NONE',  #9047 ) ;
#13471=DIRECTION ( 'NONE',  ( -1.000000000000000000, 0.000000000000000000, 0.000000000000000000 ) ) ;
#13513=CARTESIAN_POINT ( 'NONE',  ( 5.400000000000015454, -1.000000000000002220, -30.00000000000000000 ) ) ;
#13528=EDGE_LOOP ( 'NONE', ( #26678, #1161, #5920, #21177, #35548, #28268 ) ) ;
#13556=AXIS2_PLACEMENT_3D ( 'NONE', #8703, #19507, #14104 ) ;
#13600=LINE ( 'NONE', #13784, #12849 ) ;
#13696=CIRCLE ( 'NONE', #22283, 4.000000000000000000 ) ;
#13709=ORIENTED_EDGE ( 'NONE', *, *, #28615, .T. ) ;
#13726=VERTEX_POINT ( 'NONE', #82 ) ;
#13775=EDGE_CURVE ( 'NONE', #29301, #10171, #7638, .T. ) ;
#13776=CARTESIAN_POINT ( 'NONE',  ( -4.000000000000000000, -2.710505431213761085E-17, 55.00000000000000000 ) ) ;
#13783=CYLINDRICAL_SURFACE ( 'NONE', #34369, 3.799999999999999822 ) ;
#13784=CARTESIAN_POINT ( 'NONE',  ( 4.000000000000000000, 4.627536653468036720E-16, 55.00000000000000000 ) ) ;
#13798=DIRECTION ( 'NONE',  ( 1.000000000000000000, 0.000000000000000000, 0.000000000000000000 ) ) ;
#13801=LINE ( 'NONE', #30185, #34086 ) ;
#13872=CYLINDRICAL_SURFACE ( 'NONE', #11555, 4.000000000000000000 ) ;
#13914=ORIENTED_EDGE ( 'NONE', *, *, #29353, .F. ) ;
#13917=LINE ( 'NONE', #2959, #2821 ) ;
#13958=ORIENTED_EDGE ( 'NONE', *, *, #33503, .F. ) ;
#14020=ORIENTED_EDGE ( 'NONE', *, *, #4659, .T. ) ;
#14026=DIRECTION ( 'NONE',  ( -0.000000000000000000, 0.000000000000000000, -1.000000000000000000 ) ) ;
#14035=FACE_OUTER_BOUND ( 'NONE', #13528, .T. ) ;
#14084=EDGE_CURVE ( 'NONE', #4520, #13350, #2686, .T. ) ;
#14104=DIRECTION ( 'NONE',  ( -1.000000000000000000, 0.000000000000000000, 0.000000000000000000 ) ) ;
#14153=CARTESIAN_POINT ( 'NONE',  ( 0.000000000000000000, -2.710505431213761085E-17, 29.09999999999999787 ) ) ;
#14180=ORIENTED_EDGE ( 'NONE', *, *, #15009, .F. ) ;
#14223=ORIENTED_EDGE ( 'NONE', *, *, #15219, .T. ) ;
#14268=DIRECTION ( 'NONE',  ( -0.000000000000000000, 0.000000000000000000, -1.000000000000000000 ) ) ;
#14279=DIRECTION ( 'NONE',  ( -1.000000000000000000, 0.000000000000000000, 0.000000000000000000 ) ) ;
#14294=EDGE_LOOP ( 'NONE', ( #25915, #2638, #22160, #25773 ) ) ;
#14302=CYLINDRICAL_SURFACE ( 'NONE', #16027, 4.000000000000000000 ) ;
#14345=ORIENTED_EDGE ( 'NONE', *, *, #19007, .T. ) ;
#14361=AXIS2_PLACEMENT_3D ( 'NONE', #27191, #31293, #33625 ) ;
#14362=DIRECTION ( 'NONE',  ( 1.000000000000000000, 0.000000000000000000, 0.000000000000000000 ) ) ;
#14364=EDGE_LOOP ( 'NONE', ( #22970, #5811, #21389, #4406 ) ) ;
#14378=CARTESIAN_POINT ( 'NONE',  ( 3.799999999999999822, -2.710505431213761085E-17, -21.89999999999999858 ) ) ;
#14385=DIRECTION ( 'NONE',  ( -1.000000000000000000, 0.000000000000000000, 0.000000000000000000 ) ) ;
#14388=CIRCLE ( 'NONE', #16110, 4.000000000000000000 ) ;
#14412=CARTESIAN_POINT ( 'NONE',  ( 0.000000000000000000, -2.710505431213761085E-17, 55.00000000000000000 ) ) ;
#14446=ADVANCED_FACE ( 'NONE', ( #8182 ), #15561, .T. ) ;
#14461=ORIENTED_EDGE ( 'NONE', *, *, #8030, .F. ) ;
#14467=CIRCLE ( 'NONE', #34619, 3.799999999999999822 ) ;
#14482=CYLINDRICAL_SURFACE ( 'NONE', #32990, 3.799999999999999822 ) ;
#14490=CARTESIAN_POINT ( 'NONE',  ( 5.400000000000015454, -1.000000000000002220, 38.00000000000000000 ) ) ;
#14524=CARTESIAN_POINT ( 'NONE',  ( 0.000000000000000000, -2.710505431213761085E-17, 38.00000000000000711 ) ) ;
#14540=EDGE_LOOP ( 'NONE', ( #14786, #3501, #34504, #14797 ) ) ;
#14542=DIRECTION ( 'NONE',  ( -1.000000000000000000, 0.000000000000000000, 0.000000000000000000 ) ) ;
#14543=PLANE ( 'NONE',  #27263 ) ;
#14571=EDGE_CURVE ( 'NONE', #1603, #3820, #30692, .T. ) ;
#14576=CIRCLE ( 'NONE', #12866, 3.799999999999999822 ) ;
#14585=FACE_OUTER_BOUND ( 'NONE', #9427, .T. ) ;
#14620=DIRECTION ( 'NONE',  ( 0.000000000000000000, 0.000000000000000000, 1.000000000000000000 ) ) ;
#14633=CARTESIAN_POINT ( 'NONE',  ( 3.799999999999999822, -2.710505431213761085E-17, -45.00000000000000000 ) ) ;
#14686=CIRCLE ( 'NONE', #24485, 4.000000000000000000 ) ;
#14718=VERTEX_POINT ( 'NONE', #14633 ) ;
#14720=VECTOR ( 'NONE', #3452, 1000.000000000000000 ) ;
#14725=VERTEX_POINT ( 'NONE', #9072 ) ;
#14740=EDGE_CURVE ( 'NONE', #17196, #6339, #27402, .T. ) ;
#14783=VECTOR ( 'NONE', #4362, 1000.000000000000000 ) ;
#14786=ORIENTED_EDGE ( 'NONE', *, *, #24435, .F. ) ;
#14797=ORIENTED_EDGE ( 'NONE', *, *, #28808, .F. ) ;
#14820=FACE_OUTER_BOUND ( 'NONE', #34730, .T. ) ;
#14873=PLANE ( 'NONE',  #1459 ) ;
#14876=CARTESIAN_POINT ( 'NONE',  ( -4.000000000000000000, -2.710505431213761085E-17, 38.00000000000000711 ) ) ;
#14879=CIRCLE ( 'NONE', #33887, 3.799999999999999822 ) ;
#14925=ADVANCED_FACE ( 'NONE', ( #29414 ), #18236, .T. ) ;
#14969=DIRECTION ( 'NONE',  ( 1.000000000000000000, 0.000000000000000000, 0.000000000000000000 ) ) ;
#14970=ADVANCED_FACE ( 'NONE', ( #24188 ), #32456, .T. ) ;
#15009=EDGE_CURVE ( 'NONE', #7912, #23627, #33760, .T. ) ;
#15071=DIRECTION ( 'NONE',  ( -1.000000000000000000, 0.000000000000000000, 0.000000000000000000 ) ) ;
#15090=VECTOR ( 'NONE', #26378, 1000.000000000000000 ) ;
#15153=VERTEX_POINT ( 'NONE', #30815 ) ;
#15174=EDGE_LOOP ( 'NONE', ( #30605, #2160, #15603, #31146, #25524 ) ) ;
#15219=EDGE_CURVE ( 'NONE', #14718, #28677, #28038, .T. ) ;
#15238=EDGE_CURVE ( 'NONE', #908, #25349, #17839, .T. ) ;
#15239=FACE_OUTER_BOUND ( 'NONE', #2902, .T. ) ;
#15246=CARTESIAN_POINT ( 'NONE',  ( 4.000000000000000000, 4.627536653468036720E-16, -22.00000000000000000 ) ) ;
#15267=AXIS2_PLACEMENT_3D ( 'NONE', #29890, #3056, #11328 ) ;
#15287=DIRECTION ( 'NONE',  ( -1.000000000000000000, 0.000000000000000000, 0.000000000000000000 ) ) ;
#15295=CIRCLE ( 'NONE', #28553, 3.799999999999999822 ) ;
#15297=CYLINDRICAL_SURFACE ( 'NONE', #26252, 3.799999999999999822 ) ;
#15361=AXIS2_PLACEMENT_3D ( 'NONE', #34241, #4014, #20542 ) ;
#15369=DIRECTION ( 'NONE',  ( 0.000000000000000000, 0.000000000000000000, 1.000000000000000000 ) ) ;
#15438=VERTEX_POINT ( 'NONE', #20885 ) ;
#15447=ORIENTED_EDGE ( 'NONE', *, *, #6823, .T. ) ;
#15457=ADVANCED_FACE ( 'NONE', ( #21070 ), #27037, .T. ) ;
#15482=VERTEX_POINT ( 'NONE', #7219 ) ;
#15513=CARTESIAN_POINT ( 'NONE',  ( -4.000000000000000000, -2.710505431213761085E-17, 29.09999999999999787 ) ) ;
#15522=CARTESIAN_POINT ( 'NONE',  ( 0.000000000000000000, -2.710505431213761085E-17, 55.00000000000000000 ) ) ;
#15555=PLANE ( 'NONE',  #21014 ) ;
#15557=DIRECTION ( 'NONE',  ( -0.000000000000000000, 0.000000000000000000, -1.000000000000000000 ) ) ;
#15561=CYLINDRICAL_SURFACE ( 'NONE', #30854, 3.799999999999999822 ) ;
#15598=ORIENTED_EDGE ( 'NONE', *, *, #27389, .T. ) ;
#15603=ORIENTED_EDGE ( 'NONE', *, *, #35222, .T. ) ;
#15636=DIRECTION ( 'NONE',  ( 1.000000000000000000, 0.000000000000000000, 0.000000000000000000 ) ) ;
#15660=CARTESIAN_POINT ( 'NONE',  ( 0.000000000000000000, -2.710505431213761085E-17, -45.89999999999999858 ) ) ;
#15661=CARTESIAN_POINT ( 'NONE',  ( 4.000000000000000000, 4.627536653468036720E-16, -21.89999999999999858 ) ) ;
#15691=CARTESIAN_POINT ( 'NONE',  ( 4.000000000000000000, 4.627536653468036720E-16, 45.00000000000000000 ) ) ;
#15776=CARTESIAN_POINT ( 'NONE',  ( 4.000000000000000000, 4.627536653468036720E-16, -45.00000000000000000 ) ) ;
#15777=EDGE_LOOP ( 'NONE', ( #26986, #34757 ) ) ;
#15800=CYLINDRICAL_SURFACE ( 'NONE', #34110, 3.799999999999999822 ) ;
#15815=DIRECTION ( 'NONE',  ( 1.110223024625156540E-16, 1.000000000000000000, 0.000000000000000000 ) ) ;
#15836=CARTESIAN_POINT ( 'NONE',  ( 0.000000000000000000, -2.710505431213761085E-17, -20.99999999999999645 ) ) ;
#15841=( LENGTH_UNIT ( ) NAMED_UNIT ( * ) SI_UNIT ( .MILLI., .METRE. ) );
#15863=LINE ( 'NONE', #34993, #278 ) ;
#15869=LINE ( 'NONE', #7957, #7061 ) ;
#15886=ORIENTED_EDGE ( 'NONE', *, *, #21552, .F. ) ;
#15897=CARTESIAN_POINT ( 'NONE',  ( 0.000000000000000000, -2.710505431213761085E-17, 38.90000000000000568 ) ) ;
#15909=VECTOR ( 'NONE', #35211, 1000.000000000000000 ) ;
#15925=DIRECTION ( 'NONE',  ( 0.000000000000000000, 0.000000000000000000, 1.000000000000000000 ) ) ;
#15950=CARTESIAN_POINT ( 'NONE',  ( 0.000000000000000000, -2.710505431213761085E-17, 29.09999999999999787 ) ) ;
#16000=VERTEX_POINT ( 'NONE', #17567 ) ;
#16018=EDGE_LOOP ( 'NONE', ( #33695, #18644, #32, #23070 ) ) ;
#16020=( NAMED_UNIT ( * ) SI_UNIT ( $, .STERADIAN. ) SOLID_ANGLE_UNIT ( ) );
#16027=AXIS2_PLACEMENT_3D ( 'NONE', #991, #25125, #798 ) ;
#16031=CIRCLE ( 'NONE', #21236, 3.799999999999999822 ) ;
#16110=AXIS2_PLACEMENT_3D ( 'NONE', #17770, #3756, #22999 ) ;
#16112=DIRECTION ( 'NONE',  ( -0.000000000000000000, 0.000000000000000000, -1.000000000000000000 ) ) ;
#16128=FACE_BOUND ( 'NONE', #32188, .T. ) ;
#16157=DIRECTION ( 'NONE',  ( 1.000000000000000000, 0.000000000000000000, 0.000000000000000000 ) ) ;
#16161=ORIENTED_EDGE ( 'NONE', *, *, #28808, .T. ) ;
#16194=( NAMED_UNIT ( * ) PLANE_ANGLE_UNIT ( ) SI_UNIT ( $, .RADIAN. ) );
#16218=CARTESIAN_POINT ( 'NONE',  ( 0.000000000000000000, -2.710505431213761085E-17, 30.00000000000000000 ) ) ;
#16246=CIRCLE ( 'NONE', #8773, 4.000000000000000000 ) ;
#16260=CARTESIAN_POINT ( 'NONE',  ( 4.000000000000000000, 4.627536653468036720E-16, 55.00000000000000000 ) ) ;
#16291=CARTESIAN_POINT ( 'NONE',  ( -3.799999999999999822, 4.382607293638566128E-16, -45.89999999999999858 ) ) ;
#16294=EDGE_CURVE ( 'NONE', #22225, #21964, #13917, .T. ) ;
#16296=FACE_OUTER_BOUND ( 'NONE', #10232, .T. ) ;
#16300=ADVANCED_FACE ( 'NONE', ( #27624 ), #20000, .T. ) ;
#16322=ORIENTED_EDGE ( 'NONE', *, *, #6823, .F. ) ;
#16402=DIRECTION ( 'NONE',  ( 0.000000000000000000, 0.000000000000000000, 1.000000000000000000 ) ) ;
#16411=CIRCLE ( 'NONE', #13556, 4.000000000000000000 ) ;
#16459=PLANE ( 'NONE',  #11829 ) ;
#16542=FACE_OUTER_BOUND ( 'NONE', #31049, .T. ) ;
#16553=FACE_BOUND ( 'NONE', #3513, .T. ) ;
#16637=CARTESIAN_POINT ( 'NONE',  ( 3.799999999999999822, -2.710505431213761085E-17, -21.89999999999999858 ) ) ;
#16684=AXIS2_PLACEMENT_3D ( 'NONE', #20880, #31881, #351 ) ;
#16721=FACE_OUTER_BOUND ( 'NONE', #23628, .T. ) ;
#16743=CARTESIAN_POINT ( 'NONE',  ( 0.000000000000000000, -2.710505431213761085E-17, -30.90000000000000568 ) ) ;
#16855=AXIS2_PLACEMENT_3D ( 'NONE', #14524, #17408, #31111 ) ;
#16874=VECTOR ( 'NONE', #13064, 1000.000000000000000 ) ;
#16892=CYLINDRICAL_SURFACE ( 'NONE', #9661, 4.000000000000000000 ) ;
#16899=ORIENTED_EDGE ( 'NONE', *, *, #29338, .F. ) ;
#16943=EDGE_CURVE ( 'NONE', #20295, #15482, #3310, .T. ) ;
#16955=CIRCLE ( 'NONE', #4351, 4.000000000000000000 ) ;
#16972=ORIENTED_EDGE ( 'NONE', *, *, #35222, .F. ) ;
#16993=ORIENTED_EDGE ( 'NONE', *, *, #4506, .T. ) ;
#17032=AXIS2_PLACEMENT_3D ( 'NONE', #27508, #21724, #30197 ) ;
#17101=LINE ( 'NONE', #8823, #14720 ) ;
#17125=ADVANCED_FACE ( 'NONE', ( #34790 ), #28493, .T. ) ;
#17147=FACE_OUTER_BOUND ( 'NONE', #26271, .T. ) ;
#17150=EDGE_CURVE ( 'NONE', #1603, #13726, #16031, .T. ) ;
#17181=CARTESIAN_POINT ( 'NONE',  ( 0.000000000000000000, -2.710505431213761085E-17, -21.89999999999999858 ) ) ;
#17191=DIRECTION ( 'NONE',  ( 0.000000000000000000, 0.000000000000000000, -1.000000000000000000 ) ) ;
#17196=VERTEX_POINT ( 'NONE', #18029 ) ;
#17234=EDGE_CURVE ( 'NONE', #10152, #8438, #14879, .T. ) ;
#17267=CIRCLE ( 'NONE', #25366, 4.000000000000000000 ) ;
#17275=DIRECTION ( 'NONE',  ( 0.000000000000000000, 0.000000000000000000, -1.000000000000000000 ) ) ;
#17321=EDGE_CURVE ( 'NONE', #4520, #4231, #6833, .T. ) ;
#17344=COLOUR_RGB ( '', 0.09019608, 0.27058824, 0.51372549) ;
#17365=CIRCLE ( 'NONE', #1886, 4.000000000000000000 ) ;
#17392=LINE ( 'NONE', #12549, #9293 ) ;
#17402=LINE ( 'NONE', #9138, #5274 ) ;
#17408=DIRECTION ( 'NONE',  ( 0.000000000000000000, 0.000000000000000000, -1.000000000000000000 ) ) ;
#17456=CARTESIAN_POINT ( 'NONE',  ( 3.799999999999999822, -2.710505431213761085E-17, -45.89999999999999858 ) ) ;
#17468=DIRECTION ( 'NONE',  ( -1.000000000000000000, 0.000000000000000000, 0.000000000000000000 ) ) ;
#17506=CARTESIAN_POINT ( 'NONE',  ( -3.799999999999999822, 4.382607293638566128E-16, -30.90000000000000568 ) ) ;
#17557=VERTEX_POINT ( 'NONE', #28061 ) ;
#17558=CARTESIAN_POINT ( 'NONE',  ( -4.000000000000000000, -2.710505431213761085E-17, -45.89999999999999858 ) ) ;
#17567=CARTESIAN_POINT ( 'NONE',  ( 5.400000000000003020, 1.000000000000000888, 38.00000000000000000 ) ) ;
#17611=ORIENTED_EDGE ( 'NONE', *, *, #8995, .F. ) ;
#17650=DIRECTION ( 'NONE',  ( -0.000000000000000000, 0.000000000000000000, -1.000000000000000000 ) ) ;
#17712=ORIENTED_EDGE ( 'NONE', *, *, #23597, .T. ) ;
#17769=CARTESIAN_POINT ( 'NONE',  ( -4.000000000000000000, -2.710505431213761085E-17, -21.89999999999999858 ) ) ;
#17770=CARTESIAN_POINT ( 'NONE',  ( 0.000000000000000000, -2.710505431213761085E-17, -30.90000000000000568 ) ) ;
#17824=ORIENTED_EDGE ( 'NONE', *, *, #26381, .T. ) ;
#17839=LINE ( 'NONE', #28838, #14783 ) ;
#17866=CARTESIAN_POINT ( 'NONE',  ( 4.000000000000000000, 4.627536653468036720E-16, 55.00000000000000000 ) ) ;
#17869=ORIENTED_EDGE ( 'NONE', *, *, #6334, .T. ) ;
#17883=CIRCLE ( 'NONE', #26523, 4.000000000000000000 ) ;
#17894=APPLICATION_CONTEXT ( 'automotive_design' ) ;
#17904=ORIENTED_EDGE ( 'NONE', *, *, #25856, .F. ) ;
#17912=CARTESIAN_POINT ( 'NONE',  ( -4.000000000000000000, -2.710505431213761085E-17, 45.00000000000000000 ) ) ;
#17929=COLOUR_RGB ( '', 0.09019608, 0.27058824, 0.51372549) ;
#17952=CARTESIAN_POINT ( 'NONE',  ( -3.799999999999999822, 4.382607293638566128E-16, -45.89999999999999858 ) ) ;
#17988=EDGE_CURVE ( 'NONE', #15153, #751, #19409, .T. ) ;
#18014=CIRCLE ( 'NONE', #12272, 4.000000000000000000 ) ;
#18015=ORIENTED_EDGE ( 'NONE', *, *, #24298, .T. ) ;
#18029=CARTESIAN_POINT ( 'NONE',  ( -4.000000000000000000, -2.710505431213761085E-17, -55.00000000000000000 ) ) ;
#18050=DIRECTION ( 'NONE',  ( -1.000000000000000000, 1.110223024625156540E-16, 0.000000000000000000 ) ) ;
#18065=ADVANCED_FACE ( 'NONE', ( #22411 ), #30536, .T. ) ;
#18184=CIRCLE ( 'NONE', #4411, 3.799999999999999822 ) ;
#18235=CARTESIAN_POINT ( 'NONE',  ( 0.000000000000000000, -1.000000000000001554, -22.00000000000000000 ) ) ;
#18236=CYLINDRICAL_SURFACE ( 'NONE', #34334, 4.000000000000000000 ) ;
#18256=ADVANCED_FACE ( 'NONE', ( #19869 ), #25852, .T. ) ;
#18259=CARTESIAN_POINT ( 'NONE',  ( 6.071532165918824830E-15, 1.000000000000000000, 38.00000000000000000 ) ) ;
#18288=EDGE_CURVE ( 'NONE', #29301, #8849, #22333, .T. ) ;
#18292=DIRECTION ( 'NONE',  ( 1.000000000000000000, 0.000000000000000000, 0.000000000000000000 ) ) ;
#18420=ORIENTED_EDGE ( 'NONE', *, *, #12958, .T. ) ;
#18449=EDGE_LOOP ( 'NONE', ( #29468, #27659, #27952, #35136 ) ) ;
#18481=ORIENTED_EDGE ( 'NONE', *, *, #4182, .T. ) ;
#18484=DIRECTION ( 'NONE',  ( -1.000000000000000000, 0.000000000000000000, 0.000000000000000000 ) ) ;
#18503=CARTESIAN_POINT ( 'NONE',  ( 0.000000000000000000, -2.710505431213761085E-17, 45.89999999999999858 ) ) ;
#18530=CARTESIAN_POINT ( 'NONE',  ( 3.799999999999999822, -2.710505431213761085E-17, -20.99999999999999645 ) ) ;
#18537=DIRECTION ( 'NONE',  ( 0.000000000000000000, 0.000000000000000000, -1.000000000000000000 ) ) ;
#18572=EDGE_CURVE ( 'NONE', #1656, #440, #33858, .T. ) ;
#18605=AXIS2_PLACEMENT_3D ( 'NONE', #4479, #23355, #21186 ) ;
#18621=ORIENTED_EDGE ( 'NONE', *, *, #31686, .F. ) ;
#18644=ORIENTED_EDGE ( 'NONE', *, *, #17988, .T. ) ;
#18677=DIRECTION ( 'NONE',  ( 0.000000000000000000, 0.000000000000000000, -1.000000000000000000 ) ) ;
#18680=ORIENTED_EDGE ( 'NONE', *, *, #23139, .F. ) ;
#18704=CARTESIAN_POINT ( 'NONE',  ( 0.000000000000000000, -2.710505431213761085E-17, -21.89999999999999858 ) ) ;
#18711=AXIS2_PLACEMENT_3D ( 'NONE', #606, #21682, #5323 ) ;
#18770=VECTOR ( 'NONE', #28776, 1000.000000000000000 ) ;
#18830=DIRECTION ( 'NONE',  ( -1.000000000000000000, 0.000000000000000000, 0.000000000000000000 ) ) ;
#18839=AXIS2_PLACEMENT_3D ( 'NONE', #19837, #8874, #30506 ) ;
#18851=DIRECTION ( 'NONE',  ( -0.000000000000000000, 0.000000000000000000, -1.000000000000000000 ) ) ;
#18940=DIRECTION ( 'NONE',  ( 0.000000000000000000, 0.000000000000000000, -1.000000000000000000 ) ) ;
#18947=ORIENTED_EDGE ( 'NONE', *, *, #20850, .F. ) ;
#19007=EDGE_CURVE ( 'NONE', #17557, #8797, #13165, .T. ) ;
#19009=CIRCLE ( 'NONE', #31060, 4.000000000000000000 ) ;
#19019=CYLINDRICAL_SURFACE ( 'NONE', #24032, 4.000000000000000000 ) ;
#19037=DIRECTION ( 'NONE',  ( -1.000000000000000000, 0.000000000000000000, 0.000000000000000000 ) ) ;
#19038=CARTESIAN_POINT ( 'NONE',  ( 0.000000000000000000, -2.710505431213761085E-17, -30.90000000000000568 ) ) ;
#19049=FACE_OUTER_BOUND ( 'NONE', #34013, .T. ) ;
#19071=DIRECTION ( 'NONE',  ( 0.000000000000000000, 0.000000000000000000, -1.000000000000000000 ) ) ;
#19072=VERTEX_POINT ( 'NONE', #1383 ) ;
#19074=LINE ( 'NONE', #13513, #5637 ) ;
#19093=DIRECTION ( 'NONE',  ( -1.000000000000000000, 0.000000000000000000, 0.000000000000000000 ) ) ;
#19145=DIRECTION ( 'NONE',  ( -1.000000000000000000, 0.000000000000000000, 0.000000000000000000 ) ) ;
#19156=VERTEX_POINT ( 'NONE', #4640 ) ;
#19159=DIRECTION ( 'NONE',  ( 0.000000000000000000, 0.000000000000000000, 1.000000000000000000 ) ) ;
#19164=AXIS2_PLACEMENT_3D ( 'NONE', #24818, #5219, #16157 ) ;
#19188=DIRECTION ( 'NONE',  ( -0.000000000000000000, 0.000000000000000000, -1.000000000000000000 ) ) ;
#19232=FILL_AREA_STYLE ('',( #27363 ) ) ;
#19284=LINE ( 'NONE', #210, #28535 ) ;
#19289=ADVANCED_FACE ( 'NONE', ( #24248 ), #21510, .T. ) ;
#19351=ADVANCED_FACE ( 'NONE', ( #25661 ), #14302, .T. ) ;
#19352=VECTOR ( 'NONE', #31252, 1000.000000000000000 ) ;
#19409=CIRCLE ( 'NONE', #6764, 4.000000000000000000 ) ;
#19426=EDGE_LOOP ( 'NONE', ( #5315, #8945 ) ) ;
#19507=DIRECTION ( 'NONE',  ( 0.000000000000000000, 0.000000000000000000, -1.000000000000000000 ) ) ;
#19524=CARTESIAN_POINT ( 'NONE',  ( 0.000000000000000000, -2.710505431213761085E-17, -30.90000000000000568 ) ) ;
#19608=EDGE_LOOP ( 'NONE', ( #24178, #33160 ) ) ;
#19631=ORIENTED_EDGE ( 'NONE', *, *, #8352, .F. ) ;
#19690=FACE_OUTER_BOUND ( 'NONE', #619, .T. ) ;
#19704=LINE ( 'NONE', #20415, #22217 ) ;
#19711=LINE ( 'NONE', #30726, #880 ) ;
#19722=ORIENTED_EDGE ( 'NONE', *, *, #4659, .F. ) ;
#19829=LINE ( 'NONE', #3315, #25126 ) ;
#19837=CARTESIAN_POINT ( 'NONE',  ( 0.000000000000000000, -2.710505431213761085E-17, 45.89999999999999858 ) ) ;
#19855=VERTEX_POINT ( 'NONE', #11978 ) ;
#19869=FACE_OUTER_BOUND ( 'NONE', #33461, .T. ) ;
#19899=ORIENTED_EDGE ( 'NONE', *, *, #4028, .T. ) ;
#19942=ORIENTED_EDGE ( 'NONE', *, *, #2447, .F. ) ;
#19959=ORIENTED_EDGE ( 'NONE', *, *, #10820, .T. ) ;
#19969=CARTESIAN_POINT ( 'NONE',  ( 3.799999999999999822, 4.382607293638566128E-16, 45.89999999999999858 ) ) ;
#20000=CYLINDRICAL_SURFACE ( 'NONE', #20587, 4.000000000000000000 ) ;
#20019=CYLINDRICAL_SURFACE ( 'NONE', #4507, 4.000000000000000000 ) ;
#20023=DIRECTION ( 'NONE',  ( -0.000000000000000000, 0.000000000000000000, -1.000000000000000000 ) ) ;
#20037=PRODUCT_DEFINITION ( 'UNKNOWN', '', #10355, #11926 ) ;
#20092=DIRECTION ( 'NONE',  ( -1.000000000000000000, 0.000000000000000000, 0.000000000000000000 ) ) ;
#20094=ORIENTED_EDGE ( 'NONE', *, *, #14571, .T. ) ;
#20114=AXIS2_PLACEMENT_3D ( 'NONE', #4968, #1914, #10183 ) ;
#20122=PRODUCT_DEFINITION_SHAPE ( 'NONE', 'NONE',  #20037 ) ;
#20176=ORIENTED_EDGE ( 'NONE', *, *, #23830, .F. ) ;
#20179=VERTEX_POINT ( 'NONE', #24384 ) ;
#20185=AXIS2_PLACEMENT_3D ( 'NONE', #21607, #2389, #19093 ) ;
#20197=CARTESIAN_POINT ( 'NONE',  ( 3.872983346207416133, 1.000000000000001110, -22.00000000000000000 ) ) ;
#20219=ORIENTED_EDGE ( 'NONE', *, *, #6334, .F. ) ;
#20255=ORIENTED_EDGE ( 'NONE', *, *, #21592, .T. ) ;
#20287=LINE ( 'NONE', #17952, #18770 ) ;
#20295=VERTEX_POINT ( 'NONE', #8519 ) ;
#20415=CARTESIAN_POINT ( 'NONE',  ( -3.799999999999999822, 4.382607293638566128E-16, 38.00000000000000711 ) ) ;
#20433=DIRECTION ( 'NONE',  ( 0.000000000000000000, 0.000000000000000000, -1.000000000000000000 ) ) ;
#20542=DIRECTION ( 'NONE',  ( -1.000000000000000000, 0.000000000000000000, 0.000000000000000000 ) ) ;
#20574=DIRECTION ( 'NONE',  ( 0.000000000000000000, 0.000000000000000000, 1.000000000000000000 ) ) ;
#20587=AXIS2_PLACEMENT_3D ( 'NONE', #30493, #31007, #583 ) ;
#20589=CIRCLE ( 'NONE', #25217, 3.799999999999999822 ) ;
#20596=FACE_OUTER_BOUND ( 'NONE', #12228, .T. ) ;
#20641=CARTESIAN_POINT ( 'NONE',  ( 3.799999999999999822, -2.710505431213761085E-17, 29.09999999999999787 ) ) ;
#20714=CARTESIAN_POINT ( 'NONE',  ( 0.000000000000000000, -2.710505431213761085E-17, -20.99999999999999645 ) ) ;
#20747=DIRECTION ( 'NONE',  ( 1.000000000000000000, 0.000000000000000000, 0.000000000000000000 ) ) ;
#20838=FACE_BOUND ( 'NONE', #31243, .T. ) ;
#20850=EDGE_CURVE ( 'NONE', #8507, #342, #17883, .T. ) ;
#20862=FACE_OUTER_BOUND ( 'NONE', #8314, .T. ) ;
#20872=CARTESIAN_POINT ( 'NONE',  ( 0.000000000000000000, -2.710505431213761085E-17, 45.89999999999999858 ) ) ;
#20880=CARTESIAN_POINT ( 'NONE',  ( 0.000000000000000000, -2.710505431213761085E-17, -30.00000000000000711 ) ) ;
#20885=CARTESIAN_POINT ( 'NONE',  ( 4.000000000000000000, 4.627536653468036720E-16, 55.00000000000000000 ) ) ;
#20890=EDGE_LOOP ( 'NONE', ( #21875, #29242, #21640, #29372 ) ) ;
#20911=CARTESIAN_POINT ( 'NONE',  ( 0.000000000000000000, -2.710505431213761085E-17, 38.90000000000000568 ) ) ;
#20921=CARTESIAN_POINT ( 'NONE',  ( 0.000000000000000000, -2.710505431213761085E-17, 55.00000000000000000 ) ) ;
#20922=ORIENTED_EDGE ( 'NONE', *, *, #10573, .T. ) ;
#21006=ORIENTED_EDGE ( 'NONE', *, *, #18572, .F. ) ;
#21011=EDGE_LOOP ( 'NONE', ( #1469, #14020, #28293, #452 ) ) ;
#21014=AXIS2_PLACEMENT_3D ( 'NONE', #10534, #32486, #7472 ) ;
#21020=EDGE_CURVE ( 'NONE', #26362, #4628, #13801, .T. ) ;
#21036=AXIS2_PLACEMENT_3D ( 'NONE', #2770, #16402, #13376 ) ;
#21070=FACE_OUTER_BOUND ( 'NONE', #5899, .T. ) ;
#21120=DIRECTION ( 'NONE',  ( -1.000000000000000000, 0.000000000000000000, 0.000000000000000000 ) ) ;
#21124=VECTOR ( 'NONE', #10567, 1000.000000000000000 ) ;
#21177=ORIENTED_EDGE ( 'NONE', *, *, #2447, .T. ) ;
#21186=DIRECTION ( 'NONE',  ( -1.000000000000000000, 0.000000000000000000, 0.000000000000000000 ) ) ;
#21209=EDGE_CURVE ( 'NONE', #13101, #31834, #26193, .T. ) ;
#21211=AXIS2_PLACEMENT_3D ( 'NONE', #16743, #25043, #6480 ) ;
#21236=AXIS2_PLACEMENT_3D ( 'NONE', #4025, #29025, #12826 ) ;
#21247=ORIENTED_EDGE ( 'NONE', *, *, #8047, .T. ) ;
#21256=FILL_AREA_STYLE ('',( #5256 ) ) ;
#21307=AXIS2_PLACEMENT_3D ( 'NONE', #26589, #12725, #18292 ) ;
#21329=CARTESIAN_POINT ( 'NONE',  ( 0.000000000000000000, -2.710505431213761085E-17, -45.89999999999999858 ) ) ;
#21360=( GEOMETRIC_REPRESENTATION_CONTEXT ( 3 ) GLOBAL_UNCERTAINTY_ASSIGNED_CONTEXT ( ( #10767 ) ) GLOBAL_UNIT_ASSIGNED_CONTEXT ( ( #34242, #2019, #35150 ) ) REPRESENTATION_CONTEXT ( 'NONE', 'WORKASPACE' ) );
#21389=ORIENTED_EDGE ( 'NONE', *, *, #6811, .T. ) ;
#21415=ORIENTED_EDGE ( 'NONE', *, *, #29026, .F. ) ;
#21510=CYLINDRICAL_SURFACE ( 'NONE', #1666, 4.000000000000000000 ) ;
#21519=DIRECTION ( 'NONE',  ( -1.000000000000000000, 0.000000000000000000, 0.000000000000000000 ) ) ;
#21552=EDGE_CURVE ( 'NONE', #35587, #31214, #14576, .T. ) ;
#21556=ORIENTED_EDGE ( 'NONE', *, *, #17234, .F. ) ;
#21592=EDGE_CURVE ( 'NONE', #10152, #31214, #24919, .T. ) ;
#21600=DIRECTION ( 'NONE',  ( -0.000000000000000000, 0.000000000000000000, -1.000000000000000000 ) ) ;
#21607=CARTESIAN_POINT ( 'NONE',  ( 0.000000000000000000, -2.710505431213761085E-17, 45.00000000000000000 ) ) ;
#21630=ORIENTED_EDGE ( 'NONE', *, *, #4078, .T. ) ;
#21640=ORIENTED_EDGE ( 'NONE', *, *, #32346, .F. ) ;
#21641=AXIS2_PLACEMENT_3D ( 'NONE', #12305, #20574, #20747 ) ;
#21682=DIRECTION ( 'NONE',  ( 1.110223024625156540E-16, 1.000000000000000000, 0.000000000000000000 ) ) ;
#21684=CARTESIAN_POINT ( 'NONE',  ( 5.400000000000015454, -1.000000000000002220, 38.00000000000000000 ) ) ;
#21689=CIRCLE ( 'NONE', #22840, 3.799999999999999822 ) ;
#21691=FACE_OUTER_BOUND ( 'NONE', #2342, .T. ) ;
#21712=CARTESIAN_POINT ( 'NONE',  ( 0.000000000000000000, -2.710505431213761085E-17, 55.00000000000000000 ) ) ;
#21719=DIRECTION ( 'NONE',  ( -1.000000000000000000, 0.000000000000000000, 0.000000000000000000 ) ) ;
#21724=DIRECTION ( 'NONE',  ( 0.000000000000000000, 0.000000000000000000, -1.000000000000000000 ) ) ;
#21771=CARTESIAN_POINT ( 'NONE',  ( 0.000000000000000000, -2.710505431213761085E-17, -30.00000000000000711 ) ) ;
#21786=SURFACE_SIDE_STYLE ('',( #32255 ) ) ;
#21850=CARTESIAN_POINT ( 'NONE',  ( 0.000000000000000000, -2.710505431213761085E-17, 38.90000000000000568 ) ) ;
#21870=ORIENTED_EDGE ( 'NONE', *, *, #25819, .T. ) ;
#21875=ORIENTED_EDGE ( 'NONE', *, *, #11219, .T. ) ;
#21893=LINE ( 'NONE', #10747, #25746 ) ;
#21912=ORIENTED_EDGE ( 'NONE', *, *, #25529, .T. ) ;
#21964=VERTEX_POINT ( 'NONE', #26703 ) ;
#22004=ORIENTED_EDGE ( 'NONE', *, *, #25856, .T. ) ;
#22064=DIRECTION ( 'NONE',  ( 1.000000000000000000, 0.000000000000000000, 0.000000000000000000 ) ) ;
#22076=PLANE ( 'NONE',  #30306 ) ;
#22097=EDGE_CURVE ( 'NONE', #1656, #8278, #17101, .T. ) ;
#22102=CIRCLE ( 'NONE', #35364, 4.000000000000000000 ) ;
#22160=ORIENTED_EDGE ( 'NONE', *, *, #12085, .F. ) ;
#22185=AXIS2_PLACEMENT_3D ( 'NONE', #14153, #24804, #5713 ) ;
#22210=DIRECTION ( 'NONE',  ( -0.000000000000000000, 0.000000000000000000, -1.000000000000000000 ) ) ;
#22211=DIRECTION ( 'NONE',  ( -1.000000000000000000, 0.000000000000000000, 0.000000000000000000 ) ) ;
#22217=VECTOR ( 'NONE', #30718, 1000.000000000000000 ) ;
#22225=VERTEX_POINT ( 'NONE', #19969 ) ;
#22249=DIRECTION ( 'NONE',  ( 0.000000000000000000, 0.000000000000000000, -1.000000000000000000 ) ) ;
#22283=AXIS2_PLACEMENT_3D ( 'NONE', #28970, #3779, #23020 ) ;
#22309=CARTESIAN_POINT ( 'NONE',  ( 0.000000000000000000, -2.710505431213761085E-17, -45.00000000000000000 ) ) ;
#22333=CIRCLE ( 'NONE', #10280, 4.000000000000000000 ) ;
#22383=FACE_OUTER_BOUND ( 'NONE', #27900, .T. ) ;
#22411=FACE_OUTER_BOUND ( 'NONE', #21011, .T. ) ;
#22448=DIRECTION ( 'NONE',  ( 0.000000000000000000, 0.000000000000000000, 1.000000000000000000 ) ) ;
#22482=MANIFOLD_SOLID_BREP ( 'LPattern5', #25620 ) ;
#22552=CYLINDRICAL_SURFACE ( 'NONE', #18839, 3.799999999999999822 ) ;
#22577=AXIS2_PLACEMENT_3D ( 'NONE', #9067, #20023, #22918 ) ;
#22591=CARTESIAN_POINT ( 'NONE',  ( 3.799999999999999822, -2.710505431213761085E-17, 29.09999999999999787 ) ) ;
#22603=ORIENTED_EDGE ( 'NONE', *, *, #28219, .T. ) ;
#22779=FACE_OUTER_BOUND ( 'NONE', #7169, .T. ) ;
#22787=CIRCLE ( 'NONE', #4508, 4.000000000000000000 ) ;
#22788=ORIENTED_EDGE ( 'NONE', *, *, #24954, .F. ) ;
#22823=DIRECTION ( 'NONE',  ( 0.000000000000000000, 0.000000000000000000, 1.000000000000000000 ) ) ;
#22825=ORIENTED_EDGE ( 'NONE', *, *, #35406, .T. ) ;
#22828=ORIENTED_EDGE ( 'NONE', *, *, #12085, .T. ) ;
#22840=AXIS2_PLACEMENT_3D ( 'NONE', #24792, #27145, #117 ) ;
#22851=AXIS2_PLACEMENT_3D ( 'NONE', #13351, #21600, #7934 ) ;
#22868=ORIENTED_EDGE ( 'NONE', *, *, #2660, .T. ) ;
#22918=DIRECTION ( 'NONE',  ( -1.000000000000000000, 0.000000000000000000, 0.000000000000000000 ) ) ;
#22943=ADVANCED_FACE ( 'NONE', ( #34456 ), #28692, .T. ) ;
#22970=ORIENTED_EDGE ( 'NONE', *, *, #14084, .F. ) ;
#22999=DIRECTION ( 'NONE',  ( -1.000000000000000000, 0.000000000000000000, 0.000000000000000000 ) ) ;
#23006=CIRCLE ( 'NONE', #20114, 3.799999999999999822 ) ;
#23020=DIRECTION ( 'NONE',  ( -1.000000000000000000, 0.000000000000000000, 0.000000000000000000 ) ) ;
#23025=ORIENTED_EDGE ( 'NONE', *, *, #24954, .T. ) ;
#23069=DIRECTION ( 'NONE',  ( 0.000000000000000000, 0.000000000000000000, -1.000000000000000000 ) ) ;
#23070=ORIENTED_EDGE ( 'NONE', *, *, #19007, .F. ) ;
#23075=ORIENTED_EDGE ( 'NONE', *, *, #35406, .F. ) ;
#23081=CIRCLE ( 'NONE', #20185, 3.799999999999999822 ) ;
#23139=EDGE_CURVE ( 'NONE', #26512, #23627, #15869, .T. ) ;
#23243=DIRECTION ( 'NONE',  ( 0.000000000000000000, 1.000000000000000000, 0.000000000000000000 ) ) ;
#23283=ORIENTED_EDGE ( 'NONE', *, *, #25562, .T. ) ;
#23326=AXIS2_PLACEMENT_3D ( 'NONE', #11840, #22823, #14362 ) ;
#23355=DIRECTION ( 'NONE',  ( 0.000000000000000000, 0.000000000000000000, -1.000000000000000000 ) ) ;
#23371=ADVANCED_FACE ( 'NONE', ( #12411 ), #15800, .T. ) ;
#23430=AXIS2_PLACEMENT_3D ( 'NONE', #27212, #24150, #4554 ) ;
#23470=PLANE ( 'NONE',  #30825 ) ;
#23492=CARTESIAN_POINT ( 'NONE',  ( -3.799999999999999822, 4.382607293638566128E-16, -21.89999999999999858 ) ) ;
#23539=LINE ( 'NONE', #9683, #11898 ) ;
#23541=DIRECTION ( 'NONE',  ( 0.000000000000000000, 0.000000000000000000, -1.000000000000000000 ) ) ;
#23564=ADVANCED_FACE ( 'NONE', ( #19049, #10786 ), #7890, .T. ) ;
#23586=CARTESIAN_POINT ( 'NONE',  ( -4.000000000000000000, -2.710505431213761085E-17, 45.89999999999999858 ) ) ;
#23597=EDGE_CURVE ( 'NONE', #5410, #26512, #3073, .T. ) ;
#23603=ADVANCED_FACE ( 'NONE', ( #31103 ), #844, .F. ) ;
#23610=PLANE ( 'NONE',  #33767 ) ;
#23627=VERTEX_POINT ( 'NONE', #3566 ) ;
#23628=EDGE_LOOP ( 'NONE', ( #13709, #5173 ) ) ;
#23629=DIRECTION ( 'NONE',  ( -1.000000000000000000, 0.000000000000000000, 0.000000000000000000 ) ) ;
#23688=MECHANICAL_DESIGN_GEOMETRIC_PRESENTATION_REPRESENTATION('',(#32872),#98);
#23700=( GEOMETRIC_REPRESENTATION_CONTEXT ( 3 ) GLOBAL_UNCERTAINTY_ASSIGNED_CONTEXT ( ( #1353 ) ) GLOBAL_UNIT_ASSIGNED_CONTEXT ( ( #3538, #31070, #9104 ) ) REPRESENTATION_CONTEXT ( 'NONE', 'WORKASPACE' ) );
#23739=ORIENTED_EDGE ( 'NONE', *, *, #28661, .F. ) ;
#23747=ORIENTED_EDGE ( 'NONE', *, *, #657, .T. ) ;
#23781=AXIS2_PLACEMENT_3D ( 'NONE', #27870, #28226, #12017 ) ;
#23801=ORIENTED_EDGE ( 'NONE', *, *, #11674, .F. ) ;
#23830=EDGE_CURVE ( 'NONE', #751, #8797, #9141, .T. ) ;
#23945=CIRCLE ( 'NONE', #34879, 3.799999999999999822 ) ;
#24011=ORIENTED_EDGE ( 'NONE', *, *, #14084, .T. ) ;
#24029=ORIENTED_EDGE ( 'NONE', *, *, #6214, .T. ) ;
#24032=AXIS2_PLACEMENT_3D ( 'NONE', #21712, #19188, #13447 ) ;
#24033=EDGE_CURVE ( 'NONE', #34564, #4231, #2545, .T. ) ;
#24134=ORIENTED_EDGE ( 'NONE', *, *, #11488, .T. ) ;
#24149=FACE_BOUND ( 'NONE', #1355, .T. ) ;
#24150=DIRECTION ( 'NONE',  ( 0.000000000000000000, 0.000000000000000000, 1.000000000000000000 ) ) ;
#24178=ORIENTED_EDGE ( 'NONE', *, *, #17150, .T. ) ;
#24180=CARTESIAN_POINT ( 'NONE',  ( 5.400000000000003020, 1.000000000000000888, 38.00000000000000000 ) ) ;
#24188=FACE_OUTER_BOUND ( 'NONE', #12069, .T. ) ;
#24248=FACE_OUTER_BOUND ( 'NONE', #18449, .T. ) ;
#24298=EDGE_CURVE ( 'NONE', #4943, #14725, #960, .T. ) ;
#24353=CARTESIAN_POINT ( 'NONE',  ( -3.799999999999999822, 4.382607293638566128E-16, -20.99999999999999645 ) ) ;
#24357=DIRECTION ( 'NONE',  ( -1.000000000000000000, 0.000000000000000000, 0.000000000000000000 ) ) ;
#24361=CARTESIAN_POINT ( 'NONE',  ( 0.000000000000000000, -2.710505431213761085E-17, 45.00000000000000000 ) ) ;
#24384=CARTESIAN_POINT ( 'NONE',  ( 3.872983346207429900, -1.000000000000003553, 30.00000000000000000 ) ) ;
#24421=ORIENTED_EDGE ( 'NONE', *, *, #16294, .F. ) ;
#24430=AXIS2_PLACEMENT_3D ( 'NONE', #33458, #2886, #6094 ) ;
#24435=EDGE_CURVE ( 'NONE', #31659, #3685, #15863, .T. ) ;
#24485=AXIS2_PLACEMENT_3D ( 'NONE', #8347, #5841, #30685 ) ;
#24523=DIRECTION ( 'NONE',  ( 0.000000000000000000, 0.000000000000000000, -1.000000000000000000 ) ) ;
#24567=CIRCLE ( 'NONE', #25129, 4.000000000000000000 ) ;
#24582=CYLINDRICAL_SURFACE ( 'NONE', #6724, 4.000000000000000000 ) ;
#24584=PLANE ( 'NONE',  #8464 ) ;
#24712=DIRECTION ( 'NONE',  ( 0.000000000000000000, 0.000000000000000000, -1.000000000000000000 ) ) ;
#24758=FACE_OUTER_BOUND ( 'NONE', #6901, .T. ) ;
#24760=DIRECTION ( 'NONE',  ( -1.000000000000000000, 0.000000000000000000, 0.000000000000000000 ) ) ;
#24792=CARTESIAN_POINT ( 'NONE',  ( 0.000000000000000000, -2.710505431213761085E-17, -45.89999999999999858 ) ) ;
#24804=DIRECTION ( 'NONE',  ( 0.000000000000000000, 0.000000000000000000, -1.000000000000000000 ) ) ;
#24807=UNCERTAINTY_MEASURE_WITH_UNIT (LENGTH_MEASURE( 1.000000000000000082E-05 ), #15841, 'distance_accuracy_value', 'NONE');
#24818=CARTESIAN_POINT ( 'NONE',  ( 0.000000000000000000, 0.000000000000000000, 38.00000000000000000 ) ) ;
#24846=CARTESIAN_POINT ( 'NONE',  ( -4.000000000000000000, -2.710505431213761085E-17, -30.90000000000000568 ) ) ;
#24919=LINE ( 'NONE', #5832, #13002 ) ;
#24928=ADVANCED_FACE ( 'NONE', ( #20862, #32407 ), #10080, .T. ) ;
#24937=VECTOR ( 'NONE', #853, 1000.000000000000000 ) ;
#24954=EDGE_CURVE ( 'NONE', #32016, #12368, #8366, .T. ) ;
#24969=AXIS2_PLACEMENT_3D ( 'NONE', #19038, #18677, #13471 ) ;
#25011=ORIENTED_EDGE ( 'NONE', *, *, #22097, .T. ) ;
#25038=ADVANCED_FACE ( 'NONE', ( #10273 ), #32231, .T. ) ;
#25043=DIRECTION ( 'NONE',  ( 0.000000000000000000, 0.000000000000000000, -1.000000000000000000 ) ) ;
#25060=CARTESIAN_POINT ( 'NONE',  ( -4.000000000000000000, -2.710505431213761085E-17, 55.00000000000000000 ) ) ;
#25125=DIRECTION ( 'NONE',  ( -0.000000000000000000, 0.000000000000000000, -1.000000000000000000 ) ) ;
#25126=VECTOR ( 'NONE', #14268, 1000.000000000000000 ) ;
#25129=AXIS2_PLACEMENT_3D ( 'NONE', #28556, #12341, #6939 ) ;
#25146=DIRECTION ( 'NONE',  ( -1.000000000000000000, 0.000000000000000000, 0.000000000000000000 ) ) ;
#25163=CARTESIAN_POINT ( 'NONE',  ( 0.000000000000000000, -2.710505431213761085E-17, -22.00000000000000000 ) ) ;
#25170=CARTESIAN_POINT ( 'NONE',  ( 0.000000000000000000, -2.710505431213761085E-17, -22.00000000000000000 ) ) ;
#25175=CIRCLE ( 'NONE', #29220, 4.000000000000000000 ) ;
#25183=AXIS2_PLACEMENT_3D ( 'NONE', #462, #5696, #13798 ) ;
#25190=DIRECTION ( 'NONE',  ( -1.000000000000000000, 0.000000000000000000, 0.000000000000000000 ) ) ;
#25194=ADVANCED_FACE ( 'NONE', ( #16542, #2885 ), #33115, .F. ) ;
#25195=FACE_OUTER_BOUND ( 'NONE', #35088, .T. ) ;
#25217=AXIS2_PLACEMENT_3D ( 'NONE', #18503, #7875, #19037 ) ;
#25248=EDGE_LOOP ( 'NONE', ( #1044, #27651 ) ) ;
#25281=PLANE ( 'NONE',  #18711 ) ;
#25316=EDGE_CURVE ( 'NONE', #1317, #15438, #7238, .T. ) ;
#25340=DIRECTION ( 'NONE',  ( 0.000000000000000000, 0.000000000000000000, 1.000000000000000000 ) ) ;
#25349=VERTEX_POINT ( 'NONE', #6270 ) ;
#25366=AXIS2_PLACEMENT_3D ( 'NONE', #24361, #5284, #5112 ) ;
#25455=DIRECTION ( 'NONE',  ( 0.000000000000000000, 0.000000000000000000, -1.000000000000000000 ) ) ;
#25504=ORIENTED_EDGE ( 'NONE', *, *, #28219, .F. ) ;
#25524=ORIENTED_EDGE ( 'NONE', *, *, #30074, .F. ) ;
#25529=EDGE_CURVE ( 'NONE', #13350, #34564, #1592, .T. ) ;
#25562=EDGE_CURVE ( 'NONE', #28677, #14718, #18184, .T. ) ;
#25587=ORIENTED_EDGE ( 'NONE', *, *, #29353, .T. ) ;
#25620=CLOSED_SHELL ( 'NONE', ( #16300, #7258, #14925, #33259, #25635, #22943, #9497, #18065, #31025, #23371, #6982, #13046, #15457, #26238, #23603, #35248, #1586, #14446, #18256, #1951, #32063, #17125, #26288, #25038, #14970, #27957, #25194, #12836, #30226, #8477, #19351, #13273, #4408, #29052, #6363, #23564, #34432, #9096, #33631, #24928, #6726, #6078, #7943, #6002, #9574, #31255, #19289 ) ) ;
#25635=ADVANCED_FACE ( 'NONE', ( #30543 ), #5190, .T. ) ;
#25661=FACE_OUTER_BOUND ( 'NONE', #16018, .T. ) ;
#25667=DIRECTION ( 'NONE',  ( -0.000000000000000000, 0.000000000000000000, -1.000000000000000000 ) ) ;
#25746=VECTOR ( 'NONE', #5697, 1000.000000000000000 ) ;
#25767=VECTOR ( 'NONE', #9772, 1000.000000000000000 ) ;
#25773=ORIENTED_EDGE ( 'NONE', *, *, #8047, .F. ) ;
#25819=EDGE_CURVE ( 'NONE', #8438, #35587, #19704, .T. ) ;
#25820=CARTESIAN_POINT ( 'NONE',  ( 0.000000000000000000, -2.710505431213761085E-17, 55.00000000000000000 ) ) ;
#25824=CARTESIAN_POINT ( 'NONE',  ( 0.000000000000000000, -2.710505431213761085E-17, 29.09999999999999787 ) ) ;
#25852=CYLINDRICAL_SURFACE ( 'NONE', #7976, 4.000000000000000000 ) ;
#25856=EDGE_CURVE ( 'NONE', #26512, #5410, #15295, .T. ) ;
#25862=SURFACE_STYLE_FILL_AREA ( #19232 ) ;
#25881=DIRECTION ( 'NONE',  ( 0.000000000000000000, 0.000000000000000000, -1.000000000000000000 ) ) ;
#25915=ORIENTED_EDGE ( 'NONE', *, *, #33935, .T. ) ;
#25954=CARTESIAN_POINT ( 'NONE',  ( -3.799999999999999822, -2.710505431213761085E-17, 45.89999999999999858 ) ) ;
#25987=LINE ( 'NONE', #17866, #25767 ) ;
#26068=CARTESIAN_POINT ( 'NONE',  ( 0.000000000000000000, -2.710505431213761085E-17, 45.89999999999999858 ) ) ;
#26158=DIRECTION ( 'NONE',  ( -1.000000000000000000, 0.000000000000000000, 0.000000000000000000 ) ) ;
#26183=ORIENTED_EDGE ( 'NONE', *, *, #29239, .T. ) ;
#26193=LINE ( 'NONE', #34661, #15090 ) ;
#26238=ADVANCED_FACE ( 'NONE', ( #24758 ), #24582, .T. ) ;
#26249=DIRECTION ( 'NONE',  ( 1.000000000000000000, 0.000000000000000000, 0.000000000000000000 ) ) ;
#26252=AXIS2_PLACEMENT_3D ( 'NONE', #20872, #33081, #5711 ) ;
#26271=EDGE_LOOP ( 'NONE', ( #24421, #8263, #21247, #26489 ) ) ;
#26288=ADVANCED_FACE ( 'NONE', ( #14820 ), #9245, .F. ) ;
#26346=ORIENTED_EDGE ( 'NONE', *, *, #11674, .T. ) ;
#26362=VERTEX_POINT ( 'NONE', #20197 ) ;
#26365=AXIS2_PLACEMENT_3D ( 'NONE', #34693, #31449, #1209 ) ;
#26378=DIRECTION ( 'NONE',  ( 1.000000000000000000, -1.110223024625156540E-16, 0.000000000000000000 ) ) ;
#26379=CARTESIAN_POINT ( 'NONE',  ( 5.400000000000003020, 1.000000000000000888, -22.00000000000000000 ) ) ;
#26381=EDGE_CURVE ( 'NONE', #751, #15153, #16246, .T. ) ;
#26406=EDGE_CURVE ( 'NONE', #908, #5854, #178, .T. ) ;
#26407=CARTESIAN_POINT ( 'NONE',  ( -3.799999999999999822, 4.382607293638566128E-16, 38.90000000000000568 ) ) ;
#26420=EDGE_CURVE ( 'NONE', #5854, #26576, #31028, .T. ) ;
#26431=EDGE_CURVE ( 'NONE', #14725, #2330, #30855, .T. ) ;
#26469=CARTESIAN_POINT ( 'NONE',  ( -3.799999999999999822, 4.382607293638566128E-16, 29.09999999999999787 ) ) ;
#26489=ORIENTED_EDGE ( 'NONE', *, *, #10573, .F. ) ;
#26512=VERTEX_POINT ( 'NONE', #29194 ) ;
#26523=AXIS2_PLACEMENT_3D ( 'NONE', #26068, #31812, #18484 ) ;
#26576=VERTEX_POINT ( 'NONE', #9908 ) ;
#26589=CARTESIAN_POINT ( 'NONE',  ( 0.000000000000000000, 0.000000000000000000, 0.000000000000000000 ) ) ;
#26678=ORIENTED_EDGE ( 'NONE', *, *, #8352, .T. ) ;
#26685=ORIENTED_EDGE ( 'NONE', *, *, #18288, .T. ) ;
#26703=CARTESIAN_POINT ( 'NONE',  ( 3.799999999999999822, 4.382607293638566128E-16, 45.00000000000000000 ) ) ;
#26743=EDGE_CURVE ( 'NONE', #19072, #542, #2582, .T. ) ;
#26764=FACE_OUTER_BOUND ( 'NONE', #8144, .T. ) ;
#26820=CARTESIAN_POINT ( 'NONE',  ( 0.000000000000000000, -2.710505431213761085E-17, -30.90000000000000568 ) ) ;
#26838=CARTESIAN_POINT ( 'NONE',  ( 0.000000000000000000, -2.710505431213761085E-17, -45.89999999999999858 ) ) ;
#26855=DIRECTION ( 'NONE',  ( -1.000000000000000000, 0.000000000000000000, 0.000000000000000000 ) ) ;
#26879=CARTESIAN_POINT ( 'NONE',  ( 0.000000000000000000, -2.710505431213761085E-17, 29.09999999999999787 ) ) ;
#26945=ORIENTED_EDGE ( 'NONE', *, *, #4635, .T. ) ;
#26976=CYLINDRICAL_SURFACE ( 'NONE', #32811, 3.799999999999999822 ) ;
#26981=VERTEX_POINT ( 'NONE', #2325 ) ;
#26986=ORIENTED_EDGE ( 'NONE', *, *, #10820, .F. ) ;
#27037=CYLINDRICAL_SURFACE ( 'NONE', #22851, 4.000000000000000000 ) ;
#27094=AXIS2_PLACEMENT_3D ( 'NONE', #20714, #23069, #4016 ) ;
#27119=LINE ( 'NONE', #7483, #31308 ) ;
#27145=DIRECTION ( 'NONE',  ( 0.000000000000000000, 0.000000000000000000, -1.000000000000000000 ) ) ;
#27148=DIRECTION ( 'NONE',  ( -1.000000000000000000, 0.000000000000000000, 0.000000000000000000 ) ) ;
#27191=CARTESIAN_POINT ( 'NONE',  ( 0.000000000000000000, -2.710505431213761085E-17, -21.89999999999999858 ) ) ;
#27212=CARTESIAN_POINT ( 'NONE',  ( 0.000000000000000000, -2.710505431213761085E-17, 55.00000000000000000 ) ) ;
#27219=ORIENTED_EDGE ( 'NONE', *, *, #23139, .T. ) ;
#27263=AXIS2_PLACEMENT_3D ( 'NONE', #22309, #27731, #8975 ) ;
#27291=DIRECTION ( 'NONE',  ( 0.000000000000000000, 0.000000000000000000, 1.000000000000000000 ) ) ;
#27302=DIRECTION ( 'NONE',  ( 0.000000000000000000, 0.000000000000000000, 1.000000000000000000 ) ) ;
#27358=LINE ( 'NONE', #33285, #34717 ) ;
#27363=FILL_AREA_STYLE_COLOUR ( '', #17929 ) ;
#27389=EDGE_CURVE ( 'NONE', #8849, #19072, #19711, .T. ) ;
#27402=CIRCLE ( 'NONE', #21641, 4.000000000000000000 ) ;
#27468=DIRECTION ( 'NONE',  ( -0.000000000000000000, 0.000000000000000000, -1.000000000000000000 ) ) ;
#27477=CARTESIAN_POINT ( 'NONE',  ( 0.000000000000000000, 0.000000000000000000, 30.00000000000000000 ) ) ;
#27508=CARTESIAN_POINT ( 'NONE',  ( 0.000000000000000000, -2.710505431213761085E-17, -45.00000000000000000 ) ) ;
#27624=FACE_OUTER_BOUND ( 'NONE', #20890, .T. ) ;
#27651=ORIENTED_EDGE ( 'NONE', *, *, #7360, .T. ) ;
#27659=ORIENTED_EDGE ( 'NONE', *, *, #26406, .T. ) ;
#27731=DIRECTION ( 'NONE',  ( 0.000000000000000000, 0.000000000000000000, -1.000000000000000000 ) ) ;
#27780=CIRCLE ( 'NONE', #7630, 3.799999999999999822 ) ;
#27806=CIRCLE ( 'NONE', #13438, 3.799999999999999822 ) ;
#27841=CARTESIAN_POINT ( 'NONE',  ( -3.799999999999999822, 4.382607293638566128E-16, 30.00000000000000000 ) ) ;
#27870=CARTESIAN_POINT ( 'NONE',  ( 0.000000000000000000, -2.710505431213761085E-17, -30.90000000000000568 ) ) ;
#27900=EDGE_LOOP ( 'NONE', ( #4097, #26945, #29388, #23739 ) ) ;
#27952=ORIENTED_EDGE ( 'NONE', *, *, #26420, .T. ) ;
#27957=ADVANCED_FACE ( 'NONE', ( #1503 ), #23470, .F. ) ;
#28007=VECTOR ( 'NONE', #6402, 1000.000000000000000 ) ;
#28033=DIRECTION ( 'NONE',  ( -1.000000000000000000, 0.000000000000000000, 0.000000000000000000 ) ) ;
#28038=CIRCLE ( 'NONE', #15361, 3.799999999999999822 ) ;
#28057=CARTESIAN_POINT ( 'NONE',  ( 0.000000000000000000, -2.710505431213761085E-17, -55.00000000000000000 ) ) ;
#28061=CARTESIAN_POINT ( 'NONE',  ( 4.000000000000000000, 4.627536653468036720E-16, -20.99999999999999645 ) ) ;
#28152=DIRECTION ( 'NONE',  ( -1.000000000000000000, 0.000000000000000000, 0.000000000000000000 ) ) ;
#28178=EDGE_LOOP ( 'NONE', ( #33273, #2871 ) ) ;
#28219=EDGE_CURVE ( 'NONE', #12368, #28677, #20287, .T. ) ;
#28226=DIRECTION ( 'NONE',  ( 0.000000000000000000, 0.000000000000000000, -1.000000000000000000 ) ) ;
#28232=DIRECTION ( 'NONE',  ( 1.000000000000000000, -1.110223024625156540E-16, 0.000000000000000000 ) ) ;
#28268=ORIENTED_EDGE ( 'NONE', *, *, #27389, .F. ) ;
#28280=DIRECTION ( 'NONE',  ( 0.000000000000000000, 0.000000000000000000, 1.000000000000000000 ) ) ;
#28293=ORIENTED_EDGE ( 'NONE', *, *, #30764, .T. ) ;
#28294=CARTESIAN_POINT ( 'NONE',  ( 4.000000000000000000, 4.627536653468036720E-16, -45.89999999999999858 ) ) ;
#28309=EDGE_LOOP ( 'NONE', ( #21006, #4499 ) ) ;
#28331=DIRECTION ( 'NONE',  ( 0.000000000000000000, 1.000000000000000000, 0.000000000000000000 ) ) ;
#28427=CARTESIAN_POINT ( 'NONE',  ( 0.000000000000000000, -2.710505431213761085E-17, 55.00000000000000000 ) ) ;
#28441=PLANE ( 'NONE',  #4124 ) ;
#28493=PLANE ( 'NONE',  #32731 ) ;
#28535=VECTOR ( 'NONE', #24712, 1000.000000000000000 ) ;
#28553=AXIS2_PLACEMENT_3D ( 'NONE', #11619, #17191, #25146 ) ;
#28556=CARTESIAN_POINT ( 'NONE',  ( 0.000000000000000000, -2.710505431213761085E-17, 30.00000000000000000 ) ) ;
#28591=AXIS2_PLACEMENT_3D ( 'NONE', #30727, #11626, #28033 ) ;
#28615=EDGE_CURVE ( 'NONE', #8278, #10254, #32572, .T. ) ;
#28654=CYLINDRICAL_SURFACE ( 'NONE', #35462, 4.000000000000000000 ) ;
#28661=EDGE_CURVE ( 'NONE', #15482, #2330, #11621, .T. ) ;
#28677=VERTEX_POINT ( 'NONE', #3905 ) ;
#28679=DIRECTION ( 'NONE',  ( 0.000000000000000000, 0.000000000000000000, 1.000000000000000000 ) ) ;
#28692=CYLINDRICAL_SURFACE ( 'NONE', #32951, 3.799999999999999822 ) ;
#28726=DIRECTION ( 'NONE',  ( 1.000000000000000000, -1.110223024625156540E-16, 0.000000000000000000 ) ) ;
#28745=CARTESIAN_POINT ( 'NONE',  ( 5.400000000000003020, 1.000000000000000888, 30.00000000000000000 ) ) ;
#28766=EDGE_CURVE ( 'NONE', #4943, #16000, #3542, .T. ) ;
#28776=DIRECTION ( 'NONE',  ( 0.000000000000000000, 0.000000000000000000, 1.000000000000000000 ) ) ;
#28808=EDGE_CURVE ( 'NONE', #3685, #15482, #24567, .T. ) ;
#28810=CARTESIAN_POINT ( 'NONE',  ( -4.000000000000000000, -2.710505431213761085E-17, 30.00000000000000000 ) ) ;
#28838=CARTESIAN_POINT ( 'NONE',  ( 4.000000000000000000, 4.627536653468036720E-16, 55.00000000000000000 ) ) ;
#28897=CIRCLE ( 'NONE', #34643, 3.799999999999999822 ) ;
#28970=CARTESIAN_POINT ( 'NONE',  ( 0.000000000000000000, -2.710505431213761085E-17, -45.00000000000000000 ) ) ;
#28973=FACE_OUTER_BOUND ( 'NONE', #30441, .T. ) ;
#29006=ORIENTED_EDGE ( 'NONE', *, *, #9713, .T. ) ;
#29025=DIRECTION ( 'NONE',  ( 0.000000000000000000, 0.000000000000000000, -1.000000000000000000 ) ) ;
#29026=EDGE_CURVE ( 'NONE', #1317, #8507, #30157, .T. ) ;
#29052=ADVANCED_FACE ( 'NONE', ( #3151 ), #24584, .F. ) ;
#29070=AXIS2_PLACEMENT_3D ( 'NONE', #1816, #1636, #31864 ) ;
#29147=EDGE_LOOP ( 'NONE', ( #26183, #14345 ) ) ;
#29162=DIRECTION ( 'NONE',  ( 0.000000000000000000, 0.000000000000000000, -1.000000000000000000 ) ) ;
#29194=CARTESIAN_POINT ( 'NONE',  ( 3.799999999999999822, -2.710505431213761085E-17, -30.90000000000000568 ) ) ;
#29217=ORIENTED_EDGE ( 'NONE', *, *, #28766, .T. ) ;
#29220=AXIS2_PLACEMENT_3D ( 'NONE', #20911, #31908, #26158 ) ;
#29239=EDGE_CURVE ( 'NONE', #8797, #17557, #30903, .T. ) ;
#29241=DIRECTION ( 'NONE',  ( -0.000000000000000000, 0.000000000000000000, -1.000000000000000000 ) ) ;
#29242=ORIENTED_EDGE ( 'NONE', *, *, #15238, .T. ) ;
#29271=EDGE_LOOP ( 'NONE', ( #31399, #15886 ) ) ;
#29301=VERTEX_POINT ( 'NONE', #15661 ) ;
#29313=DIRECTION ( 'NONE',  ( -0.000000000000000000, 0.000000000000000000, -1.000000000000000000 ) ) ;
#29338=EDGE_CURVE ( 'NONE', #15438, #1317, #3318, .T. ) ;
#29353=EDGE_CURVE ( 'NONE', #440, #10254, #29559, .T. ) ;
#29360=CYLINDRICAL_SURFACE ( 'NONE', #4418, 3.799999999999999822 ) ;
#29372=ORIENTED_EDGE ( 'NONE', *, *, #26420, .F. ) ;
#29388=ORIENTED_EDGE ( 'NONE', *, *, #6680, .T. ) ;
#29407=DIRECTION ( 'NONE',  ( 0.000000000000000000, 0.000000000000000000, 1.000000000000000000 ) ) ;
#29413=DIRECTION ( 'NONE',  ( 1.110223024625156540E-16, 1.000000000000000000, 0.000000000000000000 ) ) ;
#29414=FACE_OUTER_BOUND ( 'NONE', #8360, .T. ) ;
#29438=MECHANICAL_DESIGN_GEOMETRIC_PRESENTATION_REPRESENTATION('',(#3582),#23700);
#29468=ORIENTED_EDGE ( 'NONE', *, *, #15238, .F. ) ;
#29502=ORIENTED_EDGE ( 'NONE', *, *, #13775, .F. ) ;
#29555=ORIENTED_EDGE ( 'NONE', *, *, #21592, .F. ) ;
#29559=LINE ( 'NONE', #32598, #1589 ) ;
#29594=DIRECTION ( 'NONE',  ( -1.000000000000000000, 0.000000000000000000, 0.000000000000000000 ) ) ;
#29602=EDGE_CURVE ( 'NONE', #10254, #8278, #13696, .T. ) ;
#29610=AXIS2_PLACEMENT_3D ( 'NONE', #21771, #19071, #15071 ) ;
#29644=AXIS2_PLACEMENT_3D ( 'NONE', #26838, #18537, #15287 ) ;
#29686=VECTOR ( 'NONE', #34714, 1000.000000000000000 ) ;
#29723=DIRECTION ( 'NONE',  ( 0.000000000000000000, 1.000000000000000000, 0.000000000000000000 ) ) ;
#29730=DIRECTION ( 'NONE',  ( 0.000000000000000000, 0.000000000000000000, -1.000000000000000000 ) ) ;
#29824=DIRECTION ( 'NONE',  ( -0.000000000000000000, 0.000000000000000000, -1.000000000000000000 ) ) ;
#29890=CARTESIAN_POINT ( 'NONE',  ( 0.000000000000000000, 0.000000000000000000, -30.00000000000000000 ) ) ;
#30066=VECTOR ( 'NONE', #33727, 1000.000000000000000 ) ;
#30074=EDGE_CURVE ( 'NONE', #10171, #26362, #8920, .T. ) ;
#30154=CARTESIAN_POINT ( 'NONE',  ( 0.000000000000000000, -2.710505431213761085E-17, 55.00000000000000000 ) ) ;
#30157=LINE ( 'NONE', #13776, #32603 ) ;
#30185=CARTESIAN_POINT ( 'NONE',  ( 6.071532165918824830E-15, 1.000000000000000000, -22.00000000000000000 ) ) ;
#30197=DIRECTION ( 'NONE',  ( -1.000000000000000000, 0.000000000000000000, 0.000000000000000000 ) ) ;
#30226=ADVANCED_FACE ( 'NONE', ( #12861, #9125 ), #14873, .T. ) ;
#30231=EDGE_CURVE ( 'NONE', #31659, #20295, #16955, .T. ) ;
#30278=CARTESIAN_POINT ( 'NONE',  ( 5.400000000000003020, 1.000000000000000888, -30.00000000000000000 ) ) ;
#30301=AXIS2_PLACEMENT_3D ( 'NONE', #20921, #10136, #4585 ) ;
#30306=AXIS2_PLACEMENT_3D ( 'NONE', #11277, #22249, #21719 ) ;
#30351=DIRECTION ( 'NONE',  ( -0.000000000000000000, 0.000000000000000000, -1.000000000000000000 ) ) ;
#30414=DIRECTION ( 'NONE',  ( 0.000000000000000000, 0.000000000000000000, -1.000000000000000000 ) ) ;
#30441=EDGE_LOOP ( 'NONE', ( #34762, #1972 ) ) ;
#30493=CARTESIAN_POINT ( 'NONE',  ( 0.000000000000000000, -2.710505431213761085E-17, 55.00000000000000000 ) ) ;
#30506=DIRECTION ( 'NONE',  ( -1.000000000000000000, 0.000000000000000000, 0.000000000000000000 ) ) ;
#30530=CIRCLE ( 'NONE', #27094, 3.799999999999999822 ) ;
#30536=CYLINDRICAL_SURFACE ( 'NONE', #25183, 3.799999999999999822 ) ;
#30541=FACE_OUTER_BOUND ( 'NONE', #11040, .T. ) ;
#30543=FACE_OUTER_BOUND ( 'NONE', #35266, .T. ) ;
#30605=ORIENTED_EDGE ( 'NONE', *, *, #2171, .F. ) ;
#30611=ORIENTED_EDGE ( 'NONE', *, *, #4035, .T. ) ;
#30685=DIRECTION ( 'NONE',  ( 1.000000000000000000, 0.000000000000000000, 0.000000000000000000 ) ) ;
#30692=LINE ( 'NONE', #16637, #2124 ) ;
#30718=DIRECTION ( 'NONE',  ( 0.000000000000000000, 0.000000000000000000, 1.000000000000000000 ) ) ;
#30726=CARTESIAN_POINT ( 'NONE',  ( -4.000000000000000000, -2.710505431213761085E-17, 55.00000000000000000 ) ) ;
#30727=CARTESIAN_POINT ( 'NONE',  ( 0.000000000000000000, -2.710505431213761085E-17, 38.00000000000000711 ) ) ;
#30764=EDGE_CURVE ( 'NONE', #9927, #3820, #30530, .T. ) ;
#30786=EDGE_LOOP ( 'NONE', ( #308, #3809, #11354, #18015 ) ) ;
#30815=CARTESIAN_POINT ( 'NONE',  ( 4.000000000000000000, 4.627536653468036720E-16, 29.09999999999999787 ) ) ;
#30816=ORIENTED_EDGE ( 'NONE', *, *, #7360, .F. ) ;
#30825=AXIS2_PLACEMENT_3D ( 'NONE', #18235, #29413, #18050 ) ;
#30854=AXIS2_PLACEMENT_3D ( 'NONE', #21329, #15925, #2103 ) ;
#30855=LINE ( 'NONE', #3502, #33508 ) ;
#30889=DIRECTION ( 'NONE',  ( 1.000000000000000000, 0.000000000000000000, 0.000000000000000000 ) ) ;
#30903=CIRCLE ( 'NONE', #9056, 4.000000000000000000 ) ;
#30974=CARTESIAN_POINT ( 'NONE',  ( 0.000000000000000000, -2.710505431213761085E-17, -21.89999999999999858 ) ) ;
#31007=DIRECTION ( 'NONE',  ( -0.000000000000000000, 0.000000000000000000, -1.000000000000000000 ) ) ;
#31025=ADVANCED_FACE ( 'NONE', ( #14035 ), #13872, .T. ) ;
#31028=LINE ( 'NONE', #8878, #13399 ) ;
#31049=EDGE_LOOP ( 'NONE', ( #32101, #17869, #7579, #26346, #13958 ) ) ;
#31060=AXIS2_PLACEMENT_3D ( 'NONE', #255, #11242, #22211 ) ;
#31070=( NAMED_UNIT ( * ) PLANE_ANGLE_UNIT ( ) SI_UNIT ( $, .RADIAN. ) );
#31084=ORIENTED_EDGE ( 'NONE', *, *, #26381, .F. ) ;
#31103=FACE_OUTER_BOUND ( 'NONE', #2907, .T. ) ;
#31111=DIRECTION ( 'NONE',  ( -1.000000000000000000, 0.000000000000000000, 0.000000000000000000 ) ) ;
#31146=ORIENTED_EDGE ( 'NONE', *, *, #21020, .F. ) ;
#31169=LINE ( 'NONE', #25060, #12146 ) ;
#31206=VECTOR ( 'NONE', #2979, 1000.000000000000000 ) ;
#31214=VERTEX_POINT ( 'NONE', #9877 ) ;
#31243=EDGE_LOOP ( 'NONE', ( #22828, #20922 ) ) ;
#31252=DIRECTION ( 'NONE',  ( 0.000000000000000000, 1.000000000000000000, 0.000000000000000000 ) ) ;
#31255=ADVANCED_FACE ( 'NONE', ( #20838, #28973 ), #28441, .F. ) ;
#31293=DIRECTION ( 'NONE',  ( 0.000000000000000000, 0.000000000000000000, -1.000000000000000000 ) ) ;
#31308=VECTOR ( 'NONE', #29824, 1000.000000000000000 ) ;
#31334=ORIENTED_EDGE ( 'NONE', *, *, #8194, .T. ) ;
#31353=CARTESIAN_POINT ( 'NONE',  ( 5.400000000000015454, -1.000000000000002220, -22.00000000000000000 ) ) ;
#31399=ORIENTED_EDGE ( 'NONE', *, *, #4035, .F. ) ;
#31449=DIRECTION ( 'NONE',  ( 0.000000000000000000, 0.000000000000000000, -1.000000000000000000 ) ) ;
#31478=CARTESIAN_POINT ( 'NONE',  ( -3.799999999999999822, 4.382607293638566128E-16, -30.90000000000000568 ) ) ;
#31534=CARTESIAN_POINT ( 'NONE',  ( -4.000000000000000000, -2.710505431213761085E-17, 55.00000000000000000 ) ) ;
#31547=ORIENTED_EDGE ( 'NONE', *, *, #7663, .T. ) ;
#31659=VERTEX_POINT ( 'NONE', #14876 ) ;
#31686=EDGE_CURVE ( 'NONE', #4628, #3462, #17392, .T. ) ;
#31691=EDGE_CURVE ( 'NONE', #22225, #11561, #14467, .T. ) ;
#31787=ORIENTED_EDGE ( 'NONE', *, *, #4028, .F. ) ;
#31793=ORIENTED_EDGE ( 'NONE', *, *, #31691, .F. ) ;
#31812=DIRECTION ( 'NONE',  ( -0.000000000000000000, 0.000000000000000000, -1.000000000000000000 ) ) ;
#31834=VERTEX_POINT ( 'NONE', #4986 ) ;
#31864=DIRECTION ( 'NONE',  ( -1.000000000000000000, 0.000000000000000000, 0.000000000000000000 ) ) ;
#31881=DIRECTION ( 'NONE',  ( 0.000000000000000000, 0.000000000000000000, -1.000000000000000000 ) ) ;
#31908=DIRECTION ( 'NONE',  ( 0.000000000000000000, 0.000000000000000000, -1.000000000000000000 ) ) ;
#32016=VERTEX_POINT ( 'NONE', #8723 ) ;
#32063=ADVANCED_FACE ( 'NONE', ( #19690 ), #8202, .T. ) ;
#32101=ORIENTED_EDGE ( 'NONE', *, *, #4506, .F. ) ;
#32188=EDGE_LOOP ( 'NONE', ( #6762, #24011 ) ) ;
#32203=ORIENTED_EDGE ( 'NONE', *, *, #14740, .T. ) ;
#32225=AXIS2_PLACEMENT_3D ( 'NONE', #4260, #15557, #6940 ) ;
#32226=CIRCLE ( 'NONE', #16684, 3.799999999999999822 ) ;
#32231=PLANE ( 'NONE',  #7775 ) ;
#32255=SURFACE_STYLE_FILL_AREA ( #21256 ) ;
#32346=EDGE_CURVE ( 'NONE', #26576, #25349, #17365, .T. ) ;
#32372=FACE_OUTER_BOUND ( 'NONE', #28309, .T. ) ;
#32397=CIRCLE ( 'NONE', #16855, 4.000000000000000000 ) ;
#32403=DIRECTION ( 'NONE',  ( 0.000000000000000000, 0.000000000000000000, 1.000000000000000000 ) ) ;
#32407=FACE_BOUND ( 'NONE', #29271, .T. ) ;
#32424=VECTOR ( 'NONE', #28726, 1000.000000000000000 ) ;
#32456=CYLINDRICAL_SURFACE ( 'NONE', #30301, 4.000000000000000000 ) ;
#32486=DIRECTION ( 'NONE',  ( 0.000000000000000000, 0.000000000000000000, 1.000000000000000000 ) ) ;
#32541=FACE_BOUND ( 'NONE', #4283, .T. ) ;
#32572=CIRCLE ( 'NONE', #17032, 4.000000000000000000 ) ;
#32598=CARTESIAN_POINT ( 'NONE',  ( 4.000000000000000000, 4.627536653468036720E-16, 55.00000000000000000 ) ) ;
#32603=VECTOR ( 'NONE', #22210, 1000.000000000000000 ) ;
#32678=CARTESIAN_POINT ( 'NONE',  ( 4.000000000000000000, 4.627536653468036720E-16, 45.89999999999999858 ) ) ;
#32731=AXIS2_PLACEMENT_3D ( 'NONE', #9934, #28679, #14969 ) ;
#32781=SURFACE_STYLE_USAGE ( .BOTH. , #21786 ) ;
#32811=AXIS2_PLACEMENT_3D ( 'NONE', #9852, #1590, #26249 ) ;
#32872=STYLED_ITEM ( 'NONE', ( #12992 ), #8640 ) ;
#32908=DIRECTION ( 'NONE',  ( 1.000000000000000000, 0.000000000000000000, 0.000000000000000000 ) ) ;
#32934=SURFACE_STYLE_USAGE ( .BOTH. , #33775 ) ;
#32951=AXIS2_PLACEMENT_3D ( 'NONE', #9773, #29407, #9412 ) ;
#32990=AXIS2_PLACEMENT_3D ( 'NONE', #4249, #3534, #30889 ) ;
#33044=DIRECTION ( 'NONE',  ( 0.000000000000000000, 0.000000000000000000, 1.000000000000000000 ) ) ;
#33081=DIRECTION ( 'NONE',  ( 0.000000000000000000, 0.000000000000000000, -1.000000000000000000 ) ) ;
#33115=PLANE ( 'NONE',  #15267 ) ;
#33118=AXIS2_PLACEMENT_3D ( 'NONE', #2281, #7641, #12707 ) ;
#33155=AXIS2_PLACEMENT_3D ( 'NONE', #13288, #18851, #27148 ) ;
#33160=ORIENTED_EDGE ( 'NONE', *, *, #628, .T. ) ;
#33210=DIRECTION ( 'NONE',  ( -1.000000000000000000, 0.000000000000000000, 0.000000000000000000 ) ) ;
#33259=ADVANCED_FACE ( 'NONE', ( #26764 ), #13783, .T. ) ;
#33273=ORIENTED_EDGE ( 'NONE', *, *, #35324, .F. ) ;
#33285=CARTESIAN_POINT ( 'NONE',  ( 0.000000000000000000, -1.000000000000001554, 30.00000000000000000 ) ) ;
#33300=EDGE_LOOP ( 'NONE', ( #31084, #2556 ) ) ;
#33349=ORIENTED_EDGE ( 'NONE', *, *, #21020, .T. ) ;
#33458=CARTESIAN_POINT ( 'NONE',  ( 0.000000000000000000, -2.710505431213761085E-17, -45.89999999999999858 ) ) ;
#33461=EDGE_LOOP ( 'NONE', ( #13914, #18420, #25011, #8228 ) ) ;
#33503=EDGE_CURVE ( 'NONE', #19156, #3462, #19074, .T. ) ;
#33508=VECTOR ( 'NONE', #28331, 1000.000000000000000 ) ;
#33564=ORIENTED_EDGE ( 'NONE', *, *, #29239, .F. ) ;
#33588=CARTESIAN_POINT ( 'NONE',  ( 6.071532165918824830E-15, 1.000000000000000000, 30.00000000000000000 ) ) ;
#33625=DIRECTION ( 'NONE',  ( -1.000000000000000000, 0.000000000000000000, 0.000000000000000000 ) ) ;
#33631=ADVANCED_FACE ( 'NONE', ( #8793 ), #16892, .T. ) ;
#33695=ORIENTED_EDGE ( 'NONE', *, *, #2660, .F. ) ;
#33727=DIRECTION ( 'NONE',  ( 1.000000000000000000, -1.110223024625156540E-16, 0.000000000000000000 ) ) ;
#33760=CIRCLE ( 'NONE', #9029, 3.799999999999999822 ) ;
#33767=AXIS2_PLACEMENT_3D ( 'NONE', #15660, #4553, #10290 ) ;
#33775=SURFACE_SIDE_STYLE ('',( #25862 ) ) ;
#33804=EDGE_LOOP ( 'NONE', ( #23075, #14180 ) ) ;
#33858=CIRCLE ( 'NONE', #21211, 4.000000000000000000 ) ;
#33887=AXIS2_PLACEMENT_3D ( 'NONE', #7231, #1480, #23629 ) ;
#33911=DIRECTION ( 'NONE',  ( -0.000000000000000000, 0.000000000000000000, -1.000000000000000000 ) ) ;
#33935=EDGE_CURVE ( 'NONE', #11561, #22225, #20589, .T. ) ;
#33949=LINE ( 'NONE', #9276, #32424 ) ;
#33980=CARTESIAN_POINT ( 'NONE',  ( 0.000000000000000000, -2.710505431213761085E-17, -20.99999999999999645 ) ) ;
#34013=EDGE_LOOP ( 'NONE', ( #34431, #825, #7712, #5330, #29217 ) ) ;
#34086=VECTOR ( 'NONE', #2313, 1000.000000000000000 ) ;
#34110=AXIS2_PLACEMENT_3D ( 'NONE', #26820, #34204, #4151 ) ;
#34204=DIRECTION ( 'NONE',  ( 0.000000000000000000, 0.000000000000000000, 1.000000000000000000 ) ) ;
#34241=CARTESIAN_POINT ( 'NONE',  ( 0.000000000000000000, -2.710505431213761085E-17, -45.00000000000000000 ) ) ;
#34242=( LENGTH_UNIT ( ) NAMED_UNIT ( * ) SI_UNIT ( .MILLI., .METRE. ) );
#34334=AXIS2_PLACEMENT_3D ( 'NONE', #15522, #29241, #29594 ) ;
#34369=AXIS2_PLACEMENT_3D ( 'NONE', #11082, #33044, #2109 ) ;
#34431=ORIENTED_EDGE ( 'NONE', *, *, #4635, .F. ) ;
#34432=ADVANCED_FACE ( 'NONE', ( #21691, #7482 ), #16459, .F. ) ;
#34456=FACE_OUTER_BOUND ( 'NONE', #14364, .T. ) ;
#34504=ORIENTED_EDGE ( 'NONE', *, *, #16943, .T. ) ;
#34564=VERTEX_POINT ( 'NONE', #8542 ) ;
#34619=AXIS2_PLACEMENT_3D ( 'NONE', #4108, #3928, #20092 ) ;
#34643=AXIS2_PLACEMENT_3D ( 'NONE', #26879, #24523, #7947 ) ;
#34661=CARTESIAN_POINT ( 'NONE',  ( 0.000000000000000000, -1.000000000000001554, -22.00000000000000000 ) ) ;
#34693=CARTESIAN_POINT ( 'NONE',  ( 0.000000000000000000, -2.710505431213761085E-17, -20.99999999999999645 ) ) ;
#34714=DIRECTION ( 'NONE',  ( 0.000000000000000000, 0.000000000000000000, 1.000000000000000000 ) ) ;
#34717=VECTOR ( 'NONE', #11145, 1000.000000000000000 ) ;
#34730=EDGE_LOOP ( 'NONE', ( #500, #18621, #16972, #15447 ) ) ;
#34757=ORIENTED_EDGE ( 'NONE', *, *, #5293, .F. ) ;
#34762=ORIENTED_EDGE ( 'NONE', *, *, #11219, .F. ) ;
#34790=FACE_OUTER_BOUND ( 'NONE', #15174, .T. ) ;
#34827=DIRECTION ( 'NONE',  ( -1.000000000000000000, 0.000000000000000000, 0.000000000000000000 ) ) ;
#34875=ORIENTED_EDGE ( 'NONE', *, *, #21552, .T. ) ;
#34879=AXIS2_PLACEMENT_3D ( 'NONE', #16218, #18940, #24357 ) ;
#34993=CARTESIAN_POINT ( 'NONE',  ( -4.000000000000000000, -2.710505431213761085E-17, 55.00000000000000000 ) ) ;
#35039=CARTESIAN_POINT ( 'NONE',  ( 4.000000000000000000, 4.627536653468036720E-16, -30.90000000000000568 ) ) ;
#35043=VECTOR ( 'NONE', #763, 1000.000000000000000 ) ;
#35088=EDGE_LOOP ( 'NONE', ( #19631, #7705 ) ) ;
#35096=PLANE ( 'NONE',  #24969 ) ;
#35136=ORIENTED_EDGE ( 'NONE', *, *, #9751, .F. ) ;
#35150=( NAMED_UNIT ( * ) SI_UNIT ( $, .STERADIAN. ) SOLID_ANGLE_UNIT ( ) );
#35175=DIRECTION ( 'NONE',  ( 0.000000000000000000, 0.000000000000000000, -1.000000000000000000 ) ) ;
#35211=DIRECTION ( 'NONE',  ( -0.000000000000000000, 0.000000000000000000, -1.000000000000000000 ) ) ;
#35222=EDGE_CURVE ( 'NONE', #31834, #4628, #3822, .T. ) ;
#35230=ORIENTED_EDGE ( 'NONE', *, *, #17321, .F. ) ;
#35248=ADVANCED_FACE ( 'NONE', ( #4892, #24149 ), #23610, .F. ) ;
#35250=DIRECTION ( 'NONE',  ( 1.110223024625156540E-16, 1.000000000000000000, 0.000000000000000000 ) ) ;
#35266=EDGE_LOOP ( 'NONE', ( #18481, #6698, #9374, #5413 ) ) ;
#35324=EDGE_CURVE ( 'NONE', #3820, #9927, #4642, .T. ) ;
#35344=DIRECTION ( 'NONE',  ( 0.000000000000000000, 0.000000000000000000, 1.000000000000000000 ) ) ;
#35364=AXIS2_PLACEMENT_3D ( 'NONE', #25163, #25340, #32908 ) ;
#35395=AXIS2_PLACEMENT_3D ( 'NONE', #25170, #8413, #493 ) ;
#35406=EDGE_CURVE ( 'NONE', #23627, #7912, #32226, .T. ) ;
#35462=AXIS2_PLACEMENT_3D ( 'NONE', #14412, #17650, #17468 ) ;
#35507=ORIENTED_EDGE ( 'NONE', *, *, #15219, .F. ) ;
#35548=ORIENTED_EDGE ( 'NONE', *, *, #26743, .F. ) ;
#35587=VERTEX_POINT ( 'NONE', #26407 ) ;
#35604=FACE_OUTER_BOUND ( 'NONE', #33300, .T. ) ;
ENDSEC;
END-ISO-10303-21;
